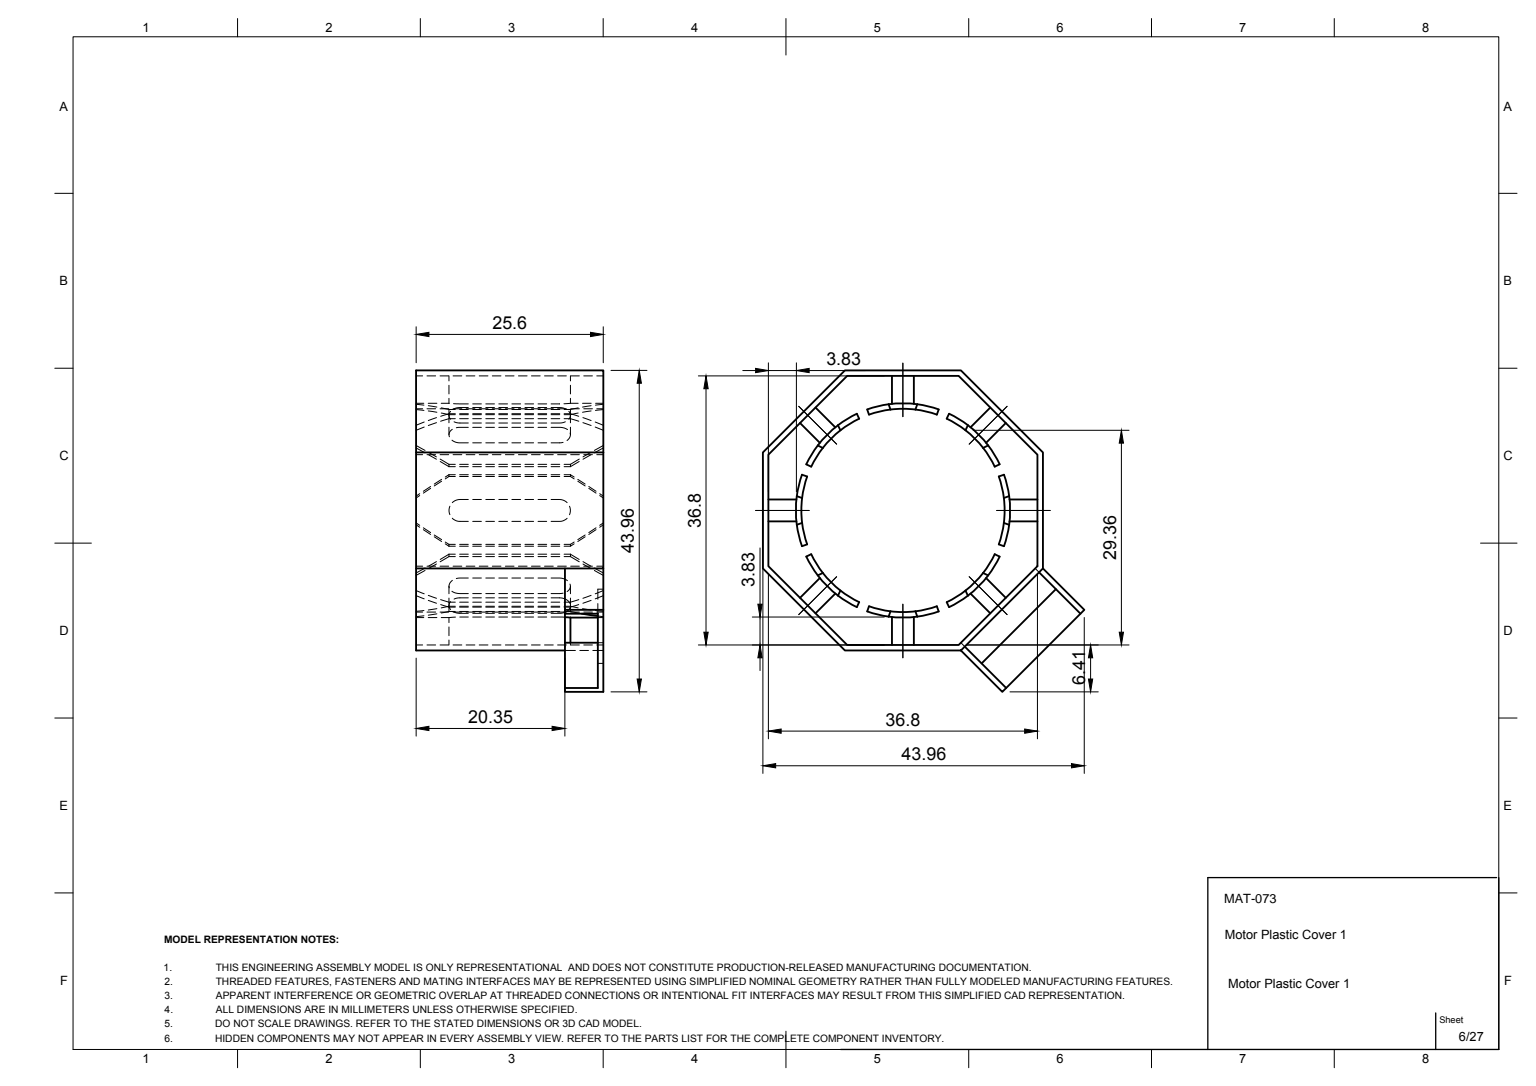
ISO-10303-21;
HEADER;
/* Generated by software containing ST-Developer
 * from STEP Tools, Inc. (www.steptools.com) 
 */

FILE_DESCRIPTION(
/* description */ ('CAx-IF Rec.Pracs.---Representation and Presentation of Product Manufa
cturing Information (PMI)---4.0---2014-10-13'),
/* implementation_level */ '2;1');

FILE_NAME(
/* name */ 'Motor Plastic Cover 1.step',
/* time_stamp */ '2026-10-24T18:52:33-07:00',
/* author */ (''),
/* organization */ (''),
/* preprocessor_version */ 'ST-DEVELOPER v20.2',
/* originating_system */ 'Autodesk Translation Framework v15.17.0.0',
/* authorisation */ '');

FILE_SCHEMA (('AP242_MANAGED_MODEL_BASED_3D_ENGINEERING_MIM_LF { 1 0 10303 442 2 1 4 }'));
ENDSEC;

DATA;
#10=MECHANICAL_DESIGN_GEOMETRIC_PRESENTATION_REPRESENTATION('',(#417),#34876);
#200=B_SPLINE_CURVE_WITH_KNOTS('',3,(#28743,#28744,#28745,#28746,#28747,
#28748,#28749,#28750,#28751,#28752,#28753,#28754,#28755,#28756,#28757,#28758,
#28759,#28760),.UNSPECIFIED.,.F.,.F.,(4,2,2,2,2,2,2,2,4),(-0.452364390465681,
-0.395818735844292,-0.339273081222902,-0.282727638227872,-0.226182195232841,
-0.16963675223781,-0.113091309242778,-0.0565456546213892,0.),
 .UNSPECIFIED.);
#201=B_SPLINE_CURVE_WITH_KNOTS('',3,(#28763,#28764,#28765,#28766,#28767,
#28768,#28769,#28770,#28771,#28772,#28773,#28774,#28775,#28776,#28777,#28778,
#28779,#28780),.UNSPECIFIED.,.F.,.F.,(4,2,2,2,2,2,2,2,4),(-0.904728780931361,
-0.848183126309972,-0.791637471688583,-0.735092028693552,-0.678546585698521,
-0.62200114270349,-0.565455699708459,-0.50891004508707,-0.452364390465681),
 .UNSPECIFIED.);
#202=B_SPLINE_CURVE_WITH_KNOTS('',3,(#28851,#28852,#28853,#28854,#28855,
#28856,#28857,#28858,#28859,#28860,#28861,#28862,#28863,#28864,#28865,#28866,
#28867,#28868),.UNSPECIFIED.,.F.,.F.,(4,2,2,2,2,2,2,2,4),(-0.452364390465681,
-0.395818735844292,-0.339273081222903,-0.282727638227872,-0.22618219523284,
-0.169636752237809,-0.113091309242778,-0.0565456546213892,0.),
 .UNSPECIFIED.);
#203=B_SPLINE_CURVE_WITH_KNOTS('',3,(#28871,#28872,#28873,#28874,#28875,
#28876,#28877,#28878,#28879,#28880,#28881,#28882,#28883,#28884,#28885,#28886,
#28887,#28888),.UNSPECIFIED.,.F.,.F.,(4,2,2,2,2,2,2,2,4),(-0.904728780931361,
-0.848183126309972,-0.791637471688583,-0.735092028693552,-0.678546585698521,
-0.622001142703489,-0.565455699708458,-0.508910045087069,-0.45236439046568),
 .UNSPECIFIED.);
#204=B_SPLINE_CURVE_WITH_KNOTS('',3,(#28959,#28960,#28961,#28962,#28963,
#28964,#28965,#28966,#28967,#28968,#28969,#28970,#28971,#28972,#28973,#28974,
#28975,#28976),.UNSPECIFIED.,.F.,.F.,(4,2,2,2,2,2,2,2,4),(-0.452364390465681,
-0.395818735844292,-0.339273081222902,-0.282727638227871,-0.22618219523284,
-0.169636752237809,-0.113091309242778,-0.0565456546213892,0.),
 .UNSPECIFIED.);
#205=B_SPLINE_CURVE_WITH_KNOTS('',3,(#28979,#28980,#28981,#28982,#28983,
#28984,#28985,#28986,#28987,#28988,#28989,#28990,#28991,#28992,#28993,#28994,
#28995,#28996),.UNSPECIFIED.,.F.,.F.,(4,2,2,2,2,2,2,2,4),(-0.904728780931362,
-0.848183126309972,-0.791637471688583,-0.735092028693552,-0.678546585698521,
-0.62200114270349,-0.565455699708459,-0.50891004508707,-0.452364390465681),
 .UNSPECIFIED.);
#206=B_SPLINE_CURVE_WITH_KNOTS('',3,(#29067,#29068,#29069,#29070,#29071,
#29072,#29073,#29074,#29075,#29076,#29077,#29078,#29079,#29080,#29081,#29082,
#29083,#29084),.UNSPECIFIED.,.F.,.F.,(4,2,2,2,2,2,2,2,4),(-0.452364390465681,
-0.395818735844292,-0.339273081222903,-0.282727638227872,-0.226182195232841,
-0.169636752237809,-0.113091309242778,-0.0565456546213892,0.),
 .UNSPECIFIED.);
#207=B_SPLINE_CURVE_WITH_KNOTS('',3,(#29087,#29088,#29089,#29090,#29091,
#29092,#29093,#29094,#29095,#29096,#29097,#29098,#29099,#29100,#29101,#29102,
#29103,#29104),.UNSPECIFIED.,.F.,.F.,(4,2,2,2,2,2,2,2,4),(-0.904728780931362,
-0.848183126309973,-0.791637471688583,-0.735092028693552,-0.678546585698521,
-0.62200114270349,-0.565455699708459,-0.50891004508707,-0.452364390465681),
 .UNSPECIFIED.);
#208=B_SPLINE_CURVE_WITH_KNOTS('',3,(#29175,#29176,#29177,#29178,#29179,
#29180,#29181,#29182,#29183,#29184,#29185,#29186,#29187,#29188,#29189,#29190,
#29191,#29192),.UNSPECIFIED.,.F.,.F.,(4,2,2,2,2,2,2,2,4),(-0.452364390465681,
-0.395818735844292,-0.339273081222903,-0.282727638227872,-0.226182195232841,
-0.169636752237809,-0.113091309242778,-0.0565456546213892,0.),
 .UNSPECIFIED.);
#209=B_SPLINE_CURVE_WITH_KNOTS('',3,(#29195,#29196,#29197,#29198,#29199,
#29200,#29201,#29202,#29203,#29204,#29205,#29206,#29207,#29208,#29209,#29210,
#29211,#29212),.UNSPECIFIED.,.F.,.F.,(4,2,2,2,2,2,2,2,4),(-0.904728780931362,
-0.848183126309973,-0.791637471688584,-0.735092028693553,-0.678546585698522,
-0.62200114270349,-0.565455699708459,-0.50891004508707,-0.452364390465681),
 .UNSPECIFIED.);
#210=B_SPLINE_CURVE_WITH_KNOTS('',3,(#29283,#29284,#29285,#29286,#29287,
#29288,#29289,#29290,#29291,#29292,#29293,#29294,#29295,#29296,#29297,#29298,
#29299,#29300),.UNSPECIFIED.,.F.,.F.,(4,2,2,2,2,2,2,2,4),(-0.452364390465681,
-0.395818735844292,-0.339273081222903,-0.282727638227872,-0.22618219523284,
-0.169636752237809,-0.113091309242778,-0.0565456546213891,0.),
 .UNSPECIFIED.);
#211=B_SPLINE_CURVE_WITH_KNOTS('',3,(#29303,#29304,#29305,#29306,#29307,
#29308,#29309,#29310,#29311,#29312,#29313,#29314,#29315,#29316,#29317,#29318,
#29319,#29320),.UNSPECIFIED.,.F.,.F.,(4,2,2,2,2,2,2,2,4),(-0.904728780931362,
-0.848183126309973,-0.791637471688583,-0.735092028693552,-0.678546585698521,
-0.62200114270349,-0.565455699708459,-0.50891004508707,-0.452364390465681),
 .UNSPECIFIED.);
#212=B_SPLINE_CURVE_WITH_KNOTS('',3,(#29391,#29392,#29393,#29394,#29395,
#29396,#29397,#29398,#29399,#29400,#29401,#29402,#29403,#29404,#29405,#29406,
#29407,#29408),.UNSPECIFIED.,.F.,.F.,(4,2,2,2,2,2,2,2,4),(-0.452364390465681,
-0.395818735844292,-0.339273081222902,-0.282727638227872,-0.226182195232841,
-0.169636752237809,-0.113091309242778,-0.0565456546213892,0.),
 .UNSPECIFIED.);
#213=B_SPLINE_CURVE_WITH_KNOTS('',3,(#29411,#29412,#29413,#29414,#29415,
#29416,#29417,#29418,#29419,#29420,#29421,#29422,#29423,#29424,#29425,#29426,
#29427,#29428),.UNSPECIFIED.,.F.,.F.,(4,2,2,2,2,2,2,2,4),(-0.904728780931362,
-0.848183126309973,-0.791637471688583,-0.735092028693552,-0.678546585698521,
-0.62200114270349,-0.565455699708459,-0.50891004508707,-0.452364390465681),
 .UNSPECIFIED.);
#214=B_SPLINE_CURVE_WITH_KNOTS('',3,(#29499,#29500,#29501,#29502,#29503,
#29504,#29505,#29506,#29507,#29508,#29509,#29510,#29511,#29512,#29513,#29514,
#29515,#29516),.UNSPECIFIED.,.F.,.F.,(4,2,2,2,2,2,2,2,4),(-0.452364390465681,
-0.395818735844292,-0.339273081222903,-0.282727638227872,-0.226182195232841,
-0.169636752237809,-0.113091309242778,-0.0565456546213892,0.),
 .UNSPECIFIED.);
#215=B_SPLINE_CURVE_WITH_KNOTS('',3,(#29519,#29520,#29521,#29522,#29523,
#29524,#29525,#29526,#29527,#29528,#29529,#29530,#29531,#29532,#29533,#29534,
#29535,#29536),.UNSPECIFIED.,.F.,.F.,(4,2,2,2,2,2,2,2,4),(-0.904728780931362,
-0.848183126309973,-0.791637471688583,-0.735092028693552,-0.678546585698521,
-0.62200114270349,-0.565455699708459,-0.50891004508707,-0.452364390465681),
 .UNSPECIFIED.);
#236=ELLIPSE('',#20061,0.0264106630927894,0.0146500000000133);
#237=ELLIPSE('',#20063,0.0264106630927895,0.0146500000000133);
#238=ELLIPSE('',#20064,0.0264106630927895,0.0146500000000133);
#239=ELLIPSE('',#20066,0.0264106630927894,0.0146500000000133);
#240=ELLIPSE('',#20069,0.0250585813644904,0.0139000000000133);
#241=ELLIPSE('',#20073,0.0250585813644904,0.0139000000000133);
#242=ELLIPSE('',#20076,0.0250585813644904,0.0139000000000133);
#243=ELLIPSE('',#20078,0.0250585813644904,0.0139000000000133);
#244=ELLIPSE('',#20089,0.0264106630927891,0.0146500000000128);
#245=ELLIPSE('',#20091,0.0264106630927891,0.0146500000000128);
#246=ELLIPSE('',#20092,0.0264106630927891,0.0146500000000128);
#247=ELLIPSE('',#20094,0.0264106630927891,0.0146500000000128);
#248=ELLIPSE('',#20097,0.0250585813644901,0.0139000000000128);
#249=ELLIPSE('',#20101,0.0250585813644901,0.0139000000000128);
#250=ELLIPSE('',#20104,0.0250585813644901,0.0139000000000128);
#251=ELLIPSE('',#20106,0.0250585813644901,0.0139000000000128);
#252=ELLIPSE('',#20117,0.0264106630927895,0.0146500000000133);
#253=ELLIPSE('',#20119,0.0264106630927894,0.0146500000000133);
#254=ELLIPSE('',#20120,0.0264106630927894,0.0146500000000133);
#255=ELLIPSE('',#20122,0.0264106630927895,0.0146500000000133);
#256=ELLIPSE('',#20125,0.0250585813644904,0.0139000000000133);
#257=ELLIPSE('',#20129,0.0250585813644904,0.0139000000000133);
#258=ELLIPSE('',#20132,0.0250585813644904,0.0139000000000133);
#259=ELLIPSE('',#20134,0.0250585813644904,0.0139000000000133);
#260=ELLIPSE('',#20145,0.0264106630927891,0.0146500000000128);
#261=ELLIPSE('',#20147,0.0264106630927891,0.0146500000000128);
#262=ELLIPSE('',#20148,0.0264106630927891,0.0146500000000128);
#263=ELLIPSE('',#20150,0.0264106630927891,0.0146500000000128);
#264=ELLIPSE('',#20153,0.0250585813644901,0.0139000000000128);
#265=ELLIPSE('',#20157,0.0250585813644901,0.0139000000000128);
#266=ELLIPSE('',#20160,0.0250585813644901,0.0139000000000128);
#267=ELLIPSE('',#20162,0.0250585813644901,0.0139000000000128);
#268=ELLIPSE('',#20173,0.0264106630927894,0.0146500000000133);
#269=ELLIPSE('',#20175,0.0264106630927895,0.0146500000000133);
#270=ELLIPSE('',#20176,0.0264106630927894,0.0146500000000133);
#271=ELLIPSE('',#20178,0.0264106630927894,0.0146500000000133);
#272=ELLIPSE('',#20181,0.0250585813644904,0.0139000000000133);
#273=ELLIPSE('',#20185,0.0250585813644904,0.0139000000000133);
#274=ELLIPSE('',#20188,0.0250585813644904,0.0139000000000133);
#275=ELLIPSE('',#20190,0.0250585813644904,0.0139000000000133);
#276=ELLIPSE('',#20201,0.0264106630927891,0.0146500000000128);
#277=ELLIPSE('',#20203,0.0264106630927891,0.0146500000000128);
#278=ELLIPSE('',#20204,0.0264106630927891,0.0146500000000128);
#279=ELLIPSE('',#20206,0.0264106630927891,0.0146500000000128);
#280=ELLIPSE('',#20209,0.0250585813644901,0.0139000000000128);
#281=ELLIPSE('',#20213,0.0250585813644901,0.0139000000000128);
#282=ELLIPSE('',#20216,0.0250585813644901,0.0139000000000128);
#283=ELLIPSE('',#20218,0.0250585813644901,0.0139000000000128);
#284=ELLIPSE('',#20229,0.0264106630927895,0.0146500000000133);
#285=ELLIPSE('',#20231,0.0264106630927894,0.0146500000000133);
#286=ELLIPSE('',#20232,0.0264106630927894,0.0146500000000133);
#287=ELLIPSE('',#20234,0.0264106630927895,0.0146500000000133);
#288=ELLIPSE('',#20237,0.0250585813644904,0.0139000000000133);
#289=ELLIPSE('',#20241,0.0250585813644904,0.0139000000000133);
#290=ELLIPSE('',#20244,0.0250585813644904,0.0139000000000133);
#291=ELLIPSE('',#20246,0.0250585813644904,0.0139000000000133);
#292=ELLIPSE('',#20257,0.0264106630927891,0.0146500000000128);
#293=ELLIPSE('',#20259,0.0264106630927891,0.0146500000000128);
#294=ELLIPSE('',#20260,0.0264106630927891,0.0146500000000128);
#295=ELLIPSE('',#20262,0.0264106630927891,0.0146500000000128);
#296=ELLIPSE('',#20265,0.0250585813644901,0.0139000000000128);
#297=ELLIPSE('',#20269,0.0250585813644901,0.0139000000000128);
#298=ELLIPSE('',#20272,0.0250585813644901,0.0139000000000128);
#299=ELLIPSE('',#20274,0.0250585813644901,0.0139000000000128);
#351=SHAPE_REPRESENTATION_RELATIONSHIP('SRR','None',#34988,#384);
#384=ADVANCED_BREP_SHAPE_REPRESENTATION('',(#450),#34846);
#417=STYLED_ITEM('',(#35162),#450);
#450=MANIFOLD_SOLID_BREP('Motor Plastic Cover 1',#19557);
#484=FACE_BOUND('',#5889,.T.);
#485=FACE_BOUND('',#5904,.T.);
#486=FACE_BOUND('',#5919,.T.);
#487=FACE_BOUND('',#5934,.T.);
#488=FACE_BOUND('',#5949,.T.);
#489=FACE_BOUND('',#5964,.T.);
#490=FACE_BOUND('',#5979,.T.);
#491=FACE_BOUND('',#5994,.T.);
#492=FACE_BOUND('',#6009,.T.);
#493=FACE_BOUND('',#6018,.T.);
#494=FACE_BOUND('',#6020,.T.);
#495=FACE_BOUND('',#6022,.T.);
#496=FACE_BOUND('',#6024,.T.);
#497=FACE_BOUND('',#6026,.T.);
#498=FACE_BOUND('',#6028,.T.);
#499=FACE_BOUND('',#6030,.T.);
#500=FACE_BOUND('',#6032,.T.);
#608=PLANE('',#20067);
#609=PLANE('',#20068);
#610=PLANE('',#20070);
#611=PLANE('',#20072);
#612=PLANE('',#20074);
#613=PLANE('',#20075);
#614=PLANE('',#20080);
#615=PLANE('',#20081);
#616=PLANE('',#20082);
#617=PLANE('',#20087);
#618=PLANE('',#20095);
#619=PLANE('',#20096);
#620=PLANE('',#20098);
#621=PLANE('',#20100);
#622=PLANE('',#20102);
#623=PLANE('',#20103);
#624=PLANE('',#20108);
#625=PLANE('',#20109);
#626=PLANE('',#20110);
#627=PLANE('',#20115);
#628=PLANE('',#20123);
#629=PLANE('',#20124);
#630=PLANE('',#20126);
#631=PLANE('',#20128);
#632=PLANE('',#20130);
#633=PLANE('',#20131);
#634=PLANE('',#20136);
#635=PLANE('',#20137);
#636=PLANE('',#20138);
#637=PLANE('',#20143);
#638=PLANE('',#20151);
#639=PLANE('',#20152);
#640=PLANE('',#20154);
#641=PLANE('',#20156);
#642=PLANE('',#20158);
#643=PLANE('',#20159);
#644=PLANE('',#20164);
#645=PLANE('',#20165);
#646=PLANE('',#20166);
#647=PLANE('',#20171);
#648=PLANE('',#20179);
#649=PLANE('',#20180);
#650=PLANE('',#20182);
#651=PLANE('',#20184);
#652=PLANE('',#20186);
#653=PLANE('',#20187);
#654=PLANE('',#20192);
#655=PLANE('',#20193);
#656=PLANE('',#20194);
#657=PLANE('',#20199);
#658=PLANE('',#20207);
#659=PLANE('',#20208);
#660=PLANE('',#20210);
#661=PLANE('',#20212);
#662=PLANE('',#20214);
#663=PLANE('',#20215);
#664=PLANE('',#20220);
#665=PLANE('',#20221);
#666=PLANE('',#20222);
#667=PLANE('',#20227);
#668=PLANE('',#20235);
#669=PLANE('',#20236);
#670=PLANE('',#20238);
#671=PLANE('',#20240);
#672=PLANE('',#20242);
#673=PLANE('',#20243);
#674=PLANE('',#20248);
#675=PLANE('',#20249);
#676=PLANE('',#20250);
#677=PLANE('',#20255);
#678=PLANE('',#20263);
#679=PLANE('',#20264);
#680=PLANE('',#20266);
#681=PLANE('',#20268);
#682=PLANE('',#20270);
#683=PLANE('',#20271);
#684=PLANE('',#20276);
#685=PLANE('',#20277);
#686=PLANE('',#20278);
#687=PLANE('',#20285);
#688=PLANE('',#20286);
#689=PLANE('',#20287);
#690=PLANE('',#20288);
#691=PLANE('',#20289);
#692=PLANE('',#20290);
#693=PLANE('',#20291);
#694=PLANE('',#20292);
#695=PLANE('',#20293);
#696=PLANE('',#20294);
#697=PLANE('',#20295);
#698=PLANE('',#20296);
#699=PLANE('',#20297);
#700=PLANE('',#20298);
#701=PLANE('',#20299);
#702=PLANE('',#20300);
#703=PLANE('',#20301);
#704=PLANE('',#20302);
#705=PLANE('',#20303);
#706=PLANE('',#20304);
#707=PLANE('',#20305);
#708=PLANE('',#20306);
#709=PLANE('',#20307);
#710=PLANE('',#20308);
#711=PLANE('',#20309);
#712=PLANE('',#20310);
#713=PLANE('',#20311);
#714=PLANE('',#20312);
#715=PLANE('',#20313);
#716=PLANE('',#20314);
#1145=LINE('',#28731,#2744);
#1146=LINE('',#28738,#2745);
#1147=LINE('',#28741,#2746);
#1148=LINE('',#28762,#2747);
#1149=LINE('',#28783,#2748);
#1150=LINE('',#28785,#2749);
#1151=LINE('',#28786,#2750);
#1152=LINE('',#28789,#2751);
#1153=LINE('',#28793,#2752);
#1154=LINE('',#28798,#2753);
#1155=LINE('',#28801,#2754);
#1156=LINE('',#28802,#2755);
#1157=LINE('',#28805,#2756);
#1158=LINE('',#28812,#2757);
#1159=LINE('',#28816,#2758);
#1160=LINE('',#28818,#2759);
#1161=LINE('',#28819,#2760);
#1162=LINE('',#28822,#2761);
#1163=LINE('',#28827,#2762);
#1164=LINE('',#28829,#2763);
#1165=LINE('',#28839,#2764);
#1166=LINE('',#28846,#2765);
#1167=LINE('',#28849,#2766);
#1168=LINE('',#28870,#2767);
#1169=LINE('',#28891,#2768);
#1170=LINE('',#28893,#2769);
#1171=LINE('',#28894,#2770);
#1172=LINE('',#28897,#2771);
#1173=LINE('',#28901,#2772);
#1174=LINE('',#28906,#2773);
#1175=LINE('',#28909,#2774);
#1176=LINE('',#28910,#2775);
#1177=LINE('',#28913,#2776);
#1178=LINE('',#28920,#2777);
#1179=LINE('',#28924,#2778);
#1180=LINE('',#28926,#2779);
#1181=LINE('',#28927,#2780);
#1182=LINE('',#28930,#2781);
#1183=LINE('',#28935,#2782);
#1184=LINE('',#28937,#2783);
#1185=LINE('',#28947,#2784);
#1186=LINE('',#28954,#2785);
#1187=LINE('',#28957,#2786);
#1188=LINE('',#28978,#2787);
#1189=LINE('',#28999,#2788);
#1190=LINE('',#29001,#2789);
#1191=LINE('',#29002,#2790);
#1192=LINE('',#29005,#2791);
#1193=LINE('',#29009,#2792);
#1194=LINE('',#29014,#2793);
#1195=LINE('',#29017,#2794);
#1196=LINE('',#29018,#2795);
#1197=LINE('',#29021,#2796);
#1198=LINE('',#29028,#2797);
#1199=LINE('',#29032,#2798);
#1200=LINE('',#29034,#2799);
#1201=LINE('',#29035,#2800);
#1202=LINE('',#29038,#2801);
#1203=LINE('',#29043,#2802);
#1204=LINE('',#29045,#2803);
#1205=LINE('',#29055,#2804);
#1206=LINE('',#29062,#2805);
#1207=LINE('',#29065,#2806);
#1208=LINE('',#29086,#2807);
#1209=LINE('',#29107,#2808);
#1210=LINE('',#29109,#2809);
#1211=LINE('',#29110,#2810);
#1212=LINE('',#29113,#2811);
#1213=LINE('',#29117,#2812);
#1214=LINE('',#29122,#2813);
#1215=LINE('',#29125,#2814);
#1216=LINE('',#29126,#2815);
#1217=LINE('',#29129,#2816);
#1218=LINE('',#29136,#2817);
#1219=LINE('',#29140,#2818);
#1220=LINE('',#29142,#2819);
#1221=LINE('',#29143,#2820);
#1222=LINE('',#29146,#2821);
#1223=LINE('',#29151,#2822);
#1224=LINE('',#29153,#2823);
#1225=LINE('',#29163,#2824);
#1226=LINE('',#29170,#2825);
#1227=LINE('',#29173,#2826);
#1228=LINE('',#29194,#2827);
#1229=LINE('',#29215,#2828);
#1230=LINE('',#29217,#2829);
#1231=LINE('',#29218,#2830);
#1232=LINE('',#29221,#2831);
#1233=LINE('',#29225,#2832);
#1234=LINE('',#29230,#2833);
#1235=LINE('',#29233,#2834);
#1236=LINE('',#29234,#2835);
#1237=LINE('',#29237,#2836);
#1238=LINE('',#29244,#2837);
#1239=LINE('',#29248,#2838);
#1240=LINE('',#29250,#2839);
#1241=LINE('',#29251,#2840);
#1242=LINE('',#29254,#2841);
#1243=LINE('',#29259,#2842);
#1244=LINE('',#29261,#2843);
#1245=LINE('',#29271,#2844);
#1246=LINE('',#29278,#2845);
#1247=LINE('',#29281,#2846);
#1248=LINE('',#29302,#2847);
#1249=LINE('',#29323,#2848);
#1250=LINE('',#29325,#2849);
#1251=LINE('',#29326,#2850);
#1252=LINE('',#29329,#2851);
#1253=LINE('',#29333,#2852);
#1254=LINE('',#29338,#2853);
#1255=LINE('',#29341,#2854);
#1256=LINE('',#29342,#2855);
#1257=LINE('',#29345,#2856);
#1258=LINE('',#29352,#2857);
#1259=LINE('',#29356,#2858);
#1260=LINE('',#29358,#2859);
#1261=LINE('',#29359,#2860);
#1262=LINE('',#29362,#2861);
#1263=LINE('',#29367,#2862);
#1264=LINE('',#29369,#2863);
#1265=LINE('',#29379,#2864);
#1266=LINE('',#29386,#2865);
#1267=LINE('',#29389,#2866);
#1268=LINE('',#29410,#2867);
#1269=LINE('',#29431,#2868);
#1270=LINE('',#29433,#2869);
#1271=LINE('',#29434,#2870);
#1272=LINE('',#29437,#2871);
#1273=LINE('',#29441,#2872);
#1274=LINE('',#29446,#2873);
#1275=LINE('',#29449,#2874);
#1276=LINE('',#29450,#2875);
#1277=LINE('',#29453,#2876);
#1278=LINE('',#29460,#2877);
#1279=LINE('',#29464,#2878);
#1280=LINE('',#29466,#2879);
#1281=LINE('',#29467,#2880);
#1282=LINE('',#29470,#2881);
#1283=LINE('',#29475,#2882);
#1284=LINE('',#29477,#2883);
#1285=LINE('',#29487,#2884);
#1286=LINE('',#29494,#2885);
#1287=LINE('',#29497,#2886);
#1288=LINE('',#29518,#2887);
#1289=LINE('',#29539,#2888);
#1290=LINE('',#29541,#2889);
#1291=LINE('',#29542,#2890);
#1292=LINE('',#29545,#2891);
#1293=LINE('',#29549,#2892);
#1294=LINE('',#29554,#2893);
#1295=LINE('',#29557,#2894);
#1296=LINE('',#29558,#2895);
#1297=LINE('',#29561,#2896);
#1298=LINE('',#29568,#2897);
#1299=LINE('',#29572,#2898);
#1300=LINE('',#29574,#2899);
#1301=LINE('',#29575,#2900);
#1302=LINE('',#29578,#2901);
#1303=LINE('',#29587,#2902);
#1304=LINE('',#29589,#2903);
#1305=LINE('',#29593,#2904);
#1306=LINE('',#29595,#2905);
#1307=LINE('',#29597,#2906);
#1308=LINE('',#29599,#2907);
#1309=LINE('',#29601,#2908);
#1310=LINE('',#29603,#2909);
#1311=LINE('',#29605,#2910);
#1312=LINE('',#29606,#2911);
#1313=LINE('',#29609,#2912);
#1314=LINE('',#29611,#2913);
#1315=LINE('',#29613,#2914);
#1316=LINE('',#29615,#2915);
#1317=LINE('',#29617,#2916);
#1318=LINE('',#29619,#2917);
#1319=LINE('',#29621,#2918);
#1320=LINE('',#29622,#2919);
#1321=LINE('',#29625,#2920);
#1322=LINE('',#29627,#2921);
#1323=LINE('',#29628,#2922);
#1324=LINE('',#29631,#2923);
#1325=LINE('',#29632,#2924);
#1326=LINE('',#29636,#2925);
#1327=LINE('',#29637,#2926);
#1328=LINE('',#29638,#2927);
#1329=LINE('',#29641,#2928);
#1330=LINE('',#29643,#2929);
#1331=LINE('',#29645,#2930);
#1332=LINE('',#29646,#2931);
#1333=LINE('',#29649,#2932);
#1334=LINE('',#29650,#2933);
#1335=LINE('',#29653,#2934);
#1336=LINE('',#29654,#2935);
#1337=LINE('',#29656,#2936);
#1338=LINE('',#29659,#2937);
#1339=LINE('',#29661,#2938);
#1340=LINE('',#29662,#2939);
#1341=LINE('',#29665,#2940);
#1342=LINE('',#29667,#2941);
#1343=LINE('',#29669,#2942);
#1344=LINE('',#29671,#2943);
#1345=LINE('',#29673,#2944);
#1346=LINE('',#29675,#2945);
#1347=LINE('',#29677,#2946);
#1348=LINE('',#29679,#2947);
#1349=LINE('',#29681,#2948);
#1350=LINE('',#29683,#2949);
#1351=LINE('',#29685,#2950);
#1352=LINE('',#29686,#2951);
#1353=LINE('',#29688,#2952);
#1354=LINE('',#29689,#2953);
#1355=LINE('',#29691,#2954);
#1356=LINE('',#29693,#2955);
#1357=LINE('',#29695,#2956);
#1358=LINE('',#29697,#2957);
#1359=LINE('',#29699,#2958);
#1360=LINE('',#29701,#2959);
#1361=LINE('',#29704,#2960);
#1362=LINE('',#29706,#2961);
#1363=LINE('',#29708,#2962);
#1364=LINE('',#29710,#2963);
#1365=LINE('',#29711,#2964);
#1366=LINE('',#29712,#2965);
#1367=LINE('',#29716,#2966);
#1368=LINE('',#29718,#2967);
#1369=LINE('',#29719,#2968);
#1370=LINE('',#29720,#2969);
#1371=LINE('',#29721,#2970);
#1372=LINE('',#29724,#2971);
#1373=LINE('',#29726,#2972);
#1374=LINE('',#29728,#2973);
#1375=LINE('',#29729,#2974);
#1376=LINE('',#29730,#2975);
#1377=LINE('',#29734,#2976);
#1378=LINE('',#29735,#2977);
#1379=LINE('',#29737,#2978);
#1380=LINE('',#29738,#2979);
#1381=LINE('',#29739,#2980);
#1382=LINE('',#29741,#2981);
#1383=LINE('',#29742,#2982);
#1384=LINE('',#29744,#2983);
#1385=LINE('',#29745,#2984);
#1386=LINE('',#29751,#2985);
#2744=VECTOR('',#22546,1.);
#2745=VECTOR('',#22553,1.);
#2746=VECTOR('',#22554,1.);
#2747=VECTOR('',#22555,1.);
#2748=VECTOR('',#22558,1.);
#2749=VECTOR('',#22559,1.);
#2750=VECTOR('',#22560,1.);
#2751=VECTOR('',#22563,1.);
#2752=VECTOR('',#22568,1.);
#2753=VECTOR('',#22575,1.);
#2754=VECTOR('',#22578,1.);
#2755=VECTOR('',#22579,1.);
#2756=VECTOR('',#22582,1.);
#2757=VECTOR('',#22593,1.);
#2758=VECTOR('',#22598,1.);
#2759=VECTOR('',#22599,1.);
#2760=VECTOR('',#22600,1.);
#2761=VECTOR('',#22603,1.);
#2762=VECTOR('',#22610,1.);
#2763=VECTOR('',#22613,1.);
#2764=VECTOR('',#22622,1.);
#2765=VECTOR('',#22629,1.);
#2766=VECTOR('',#22630,1.);
#2767=VECTOR('',#22631,1.);
#2768=VECTOR('',#22634,1.);
#2769=VECTOR('',#22635,1.);
#2770=VECTOR('',#22636,1.);
#2771=VECTOR('',#22639,1.);
#2772=VECTOR('',#22644,1.);
#2773=VECTOR('',#22651,1.);
#2774=VECTOR('',#22654,1.);
#2775=VECTOR('',#22655,1.);
#2776=VECTOR('',#22658,1.);
#2777=VECTOR('',#22669,1.);
#2778=VECTOR('',#22674,1.);
#2779=VECTOR('',#22675,1.);
#2780=VECTOR('',#22676,1.);
#2781=VECTOR('',#22679,1.);
#2782=VECTOR('',#22686,1.);
#2783=VECTOR('',#22689,1.);
#2784=VECTOR('',#22698,1.);
#2785=VECTOR('',#22705,1.);
#2786=VECTOR('',#22706,1.);
#2787=VECTOR('',#22707,1.);
#2788=VECTOR('',#22710,1.);
#2789=VECTOR('',#22711,1.);
#2790=VECTOR('',#22712,1.);
#2791=VECTOR('',#22715,1.);
#2792=VECTOR('',#22720,1.);
#2793=VECTOR('',#22727,1.);
#2794=VECTOR('',#22730,1.);
#2795=VECTOR('',#22731,1.);
#2796=VECTOR('',#22734,1.);
#2797=VECTOR('',#22745,1.);
#2798=VECTOR('',#22750,1.);
#2799=VECTOR('',#22751,1.);
#2800=VECTOR('',#22752,1.);
#2801=VECTOR('',#22755,1.);
#2802=VECTOR('',#22762,1.);
#2803=VECTOR('',#22765,1.);
#2804=VECTOR('',#22774,1.);
#2805=VECTOR('',#22781,1.);
#2806=VECTOR('',#22782,1.);
#2807=VECTOR('',#22783,1.);
#2808=VECTOR('',#22786,1.);
#2809=VECTOR('',#22787,1.);
#2810=VECTOR('',#22788,1.);
#2811=VECTOR('',#22791,1.);
#2812=VECTOR('',#22796,1.);
#2813=VECTOR('',#22803,1.);
#2814=VECTOR('',#22806,1.);
#2815=VECTOR('',#22807,1.);
#2816=VECTOR('',#22810,1.);
#2817=VECTOR('',#22821,1.);
#2818=VECTOR('',#22826,1.);
#2819=VECTOR('',#22827,1.);
#2820=VECTOR('',#22828,1.);
#2821=VECTOR('',#22831,1.);
#2822=VECTOR('',#22838,1.);
#2823=VECTOR('',#22841,1.);
#2824=VECTOR('',#22850,1.);
#2825=VECTOR('',#22857,1.);
#2826=VECTOR('',#22858,1.);
#2827=VECTOR('',#22859,1.);
#2828=VECTOR('',#22862,1.);
#2829=VECTOR('',#22863,1.);
#2830=VECTOR('',#22864,1.);
#2831=VECTOR('',#22867,1.);
#2832=VECTOR('',#22872,1.);
#2833=VECTOR('',#22879,1.);
#2834=VECTOR('',#22882,1.);
#2835=VECTOR('',#22883,1.);
#2836=VECTOR('',#22886,1.);
#2837=VECTOR('',#22897,1.);
#2838=VECTOR('',#22902,1.);
#2839=VECTOR('',#22903,1.);
#2840=VECTOR('',#22904,1.);
#2841=VECTOR('',#22907,1.);
#2842=VECTOR('',#22914,1.);
#2843=VECTOR('',#22917,1.);
#2844=VECTOR('',#22926,1.);
#2845=VECTOR('',#22933,1.);
#2846=VECTOR('',#22934,1.);
#2847=VECTOR('',#22935,1.);
#2848=VECTOR('',#22938,1.);
#2849=VECTOR('',#22939,1.);
#2850=VECTOR('',#22940,1.);
#2851=VECTOR('',#22943,1.);
#2852=VECTOR('',#22948,1.);
#2853=VECTOR('',#22955,1.);
#2854=VECTOR('',#22958,1.);
#2855=VECTOR('',#22959,1.);
#2856=VECTOR('',#22962,1.);
#2857=VECTOR('',#22973,1.);
#2858=VECTOR('',#22978,1.);
#2859=VECTOR('',#22979,1.);
#2860=VECTOR('',#22980,1.);
#2861=VECTOR('',#22983,1.);
#2862=VECTOR('',#22990,1.);
#2863=VECTOR('',#22993,1.);
#2864=VECTOR('',#23002,1.);
#2865=VECTOR('',#23009,1.);
#2866=VECTOR('',#23010,1.);
#2867=VECTOR('',#23011,1.);
#2868=VECTOR('',#23014,1.);
#2869=VECTOR('',#23015,1.);
#2870=VECTOR('',#23016,1.);
#2871=VECTOR('',#23019,1.);
#2872=VECTOR('',#23024,1.);
#2873=VECTOR('',#23031,1.);
#2874=VECTOR('',#23034,1.);
#2875=VECTOR('',#23035,1.);
#2876=VECTOR('',#23038,1.);
#2877=VECTOR('',#23049,1.);
#2878=VECTOR('',#23054,1.);
#2879=VECTOR('',#23055,1.);
#2880=VECTOR('',#23056,1.);
#2881=VECTOR('',#23059,1.);
#2882=VECTOR('',#23066,1.);
#2883=VECTOR('',#23069,1.);
#2884=VECTOR('',#23078,1.);
#2885=VECTOR('',#23085,1.);
#2886=VECTOR('',#23086,1.);
#2887=VECTOR('',#23087,1.);
#2888=VECTOR('',#23090,1.);
#2889=VECTOR('',#23091,1.);
#2890=VECTOR('',#23092,1.);
#2891=VECTOR('',#23095,1.);
#2892=VECTOR('',#23100,1.);
#2893=VECTOR('',#23107,1.);
#2894=VECTOR('',#23110,1.);
#2895=VECTOR('',#23111,1.);
#2896=VECTOR('',#23114,1.);
#2897=VECTOR('',#23125,1.);
#2898=VECTOR('',#23130,1.);
#2899=VECTOR('',#23131,1.);
#2900=VECTOR('',#23132,1.);
#2901=VECTOR('',#23135,1.);
#2902=VECTOR('',#23146,1.);
#2903=VECTOR('',#23149,1.);
#2904=VECTOR('',#23152,1.);
#2905=VECTOR('',#23153,1.);
#2906=VECTOR('',#23154,1.);
#2907=VECTOR('',#23155,1.);
#2908=VECTOR('',#23156,1.);
#2909=VECTOR('',#23157,1.);
#2910=VECTOR('',#23158,1.);
#2911=VECTOR('',#23159,1.);
#2912=VECTOR('',#23160,1.);
#2913=VECTOR('',#23161,1.);
#2914=VECTOR('',#23162,1.);
#2915=VECTOR('',#23163,1.);
#2916=VECTOR('',#23164,1.);
#2917=VECTOR('',#23165,1.);
#2918=VECTOR('',#23166,1.);
#2919=VECTOR('',#23167,1.);
#2920=VECTOR('',#23170,1.);
#2921=VECTOR('',#23171,1.);
#2922=VECTOR('',#23172,1.);
#2923=VECTOR('',#23175,1.);
#2924=VECTOR('',#23176,1.);
#2925=VECTOR('',#23179,1.);
#2926=VECTOR('',#23180,1.);
#2927=VECTOR('',#23181,1.);
#2928=VECTOR('',#23184,1.);
#2929=VECTOR('',#23185,1.);
#2930=VECTOR('',#23186,1.);
#2931=VECTOR('',#23187,1.);
#2932=VECTOR('',#23190,1.);
#2933=VECTOR('',#23191,1.);
#2934=VECTOR('',#23194,1.);
#2935=VECTOR('',#23195,1.);
#2936=VECTOR('',#23198,1.);
#2937=VECTOR('',#23201,1.);
#2938=VECTOR('',#23202,1.);
#2939=VECTOR('',#23203,1.);
#2940=VECTOR('',#23204,1.);
#2941=VECTOR('',#23205,1.);
#2942=VECTOR('',#23206,1.);
#2943=VECTOR('',#23207,1.);
#2944=VECTOR('',#23208,1.);
#2945=VECTOR('',#23209,1.);
#2946=VECTOR('',#23210,1.);
#2947=VECTOR('',#23211,1.);
#2948=VECTOR('',#23212,1.);
#2949=VECTOR('',#23213,1.);
#2950=VECTOR('',#23214,1.);
#2951=VECTOR('',#23215,1.);
#2952=VECTOR('',#23218,1.);
#2953=VECTOR('',#23219,1.);
#2954=VECTOR('',#23222,1.);
#2955=VECTOR('',#23225,1.);
#2956=VECTOR('',#23228,1.);
#2957=VECTOR('',#23231,1.);
#2958=VECTOR('',#23234,1.);
#2959=VECTOR('',#23237,1.);
#2960=VECTOR('',#23240,1.);
#2961=VECTOR('',#23241,1.);
#2962=VECTOR('',#23242,1.);
#2963=VECTOR('',#23243,1.);
#2964=VECTOR('',#23244,1.);
#2965=VECTOR('',#23245,1.);
#2966=VECTOR('',#23248,1.);
#2967=VECTOR('',#23249,1.);
#2968=VECTOR('',#23250,1.);
#2969=VECTOR('',#23251,1.);
#2970=VECTOR('',#23252,1.);
#2971=VECTOR('',#23255,1.);
#2972=VECTOR('',#23256,1.);
#2973=VECTOR('',#23257,1.);
#2974=VECTOR('',#23258,1.);
#2975=VECTOR('',#23259,1.);
#2976=VECTOR('',#23264,1.);
#2977=VECTOR('',#23265,1.);
#2978=VECTOR('',#23266,1.);
#2979=VECTOR('',#23267,1.);
#2980=VECTOR('',#23268,1.);
#2981=VECTOR('',#23271,1.);
#2982=VECTOR('',#23272,1.);
#2983=VECTOR('',#23275,1.);
#2984=VECTOR('',#23276,1.);
#2985=VECTOR('',#23287,1.);
#4307=CYLINDRICAL_SURFACE('',#20060,0.01465);
#4308=CYLINDRICAL_SURFACE('',#20077,0.0139);
#4309=CYLINDRICAL_SURFACE('',#20083,0.0015);
#4310=CYLINDRICAL_SURFACE('',#20085,0.0015);
#4311=CYLINDRICAL_SURFACE('',#20088,0.01465);
#4312=CYLINDRICAL_SURFACE('',#20105,0.0139);
#4313=CYLINDRICAL_SURFACE('',#20111,0.0015);
#4314=CYLINDRICAL_SURFACE('',#20113,0.0015);
#4315=CYLINDRICAL_SURFACE('',#20116,0.01465);
#4316=CYLINDRICAL_SURFACE('',#20133,0.0139);
#4317=CYLINDRICAL_SURFACE('',#20139,0.0015);
#4318=CYLINDRICAL_SURFACE('',#20141,0.0015);
#4319=CYLINDRICAL_SURFACE('',#20144,0.01465);
#4320=CYLINDRICAL_SURFACE('',#20161,0.0139);
#4321=CYLINDRICAL_SURFACE('',#20167,0.0015);
#4322=CYLINDRICAL_SURFACE('',#20169,0.0015);
#4323=CYLINDRICAL_SURFACE('',#20172,0.01465);
#4324=CYLINDRICAL_SURFACE('',#20189,0.0139);
#4325=CYLINDRICAL_SURFACE('',#20195,0.0015);
#4326=CYLINDRICAL_SURFACE('',#20197,0.0015);
#4327=CYLINDRICAL_SURFACE('',#20200,0.01465);
#4328=CYLINDRICAL_SURFACE('',#20217,0.0139);
#4329=CYLINDRICAL_SURFACE('',#20223,0.0015);
#4330=CYLINDRICAL_SURFACE('',#20225,0.0015);
#4331=CYLINDRICAL_SURFACE('',#20228,0.01465);
#4332=CYLINDRICAL_SURFACE('',#20245,0.0139);
#4333=CYLINDRICAL_SURFACE('',#20251,0.0015);
#4334=CYLINDRICAL_SURFACE('',#20253,0.0015);
#4335=CYLINDRICAL_SURFACE('',#20256,0.01465);
#4336=CYLINDRICAL_SURFACE('',#20273,0.0139);
#4337=CYLINDRICAL_SURFACE('',#20279,0.0015);
#4338=CYLINDRICAL_SURFACE('',#20281,0.0015);
#4839=FACE_OUTER_BOUND('',#5888,.T.);
#4840=FACE_OUTER_BOUND('',#5890,.T.);
#4841=FACE_OUTER_BOUND('',#5891,.T.);
#4842=FACE_OUTER_BOUND('',#5892,.T.);
#4843=FACE_OUTER_BOUND('',#5893,.T.);
#4844=FACE_OUTER_BOUND('',#5894,.T.);
#4845=FACE_OUTER_BOUND('',#5895,.T.);
#4846=FACE_OUTER_BOUND('',#5896,.T.);
#4847=FACE_OUTER_BOUND('',#5897,.T.);
#4848=FACE_OUTER_BOUND('',#5898,.T.);
#4849=FACE_OUTER_BOUND('',#5899,.T.);
#4850=FACE_OUTER_BOUND('',#5900,.T.);
#4851=FACE_OUTER_BOUND('',#5901,.T.);
#4852=FACE_OUTER_BOUND('',#5902,.T.);
#4853=FACE_OUTER_BOUND('',#5903,.T.);
#4854=FACE_OUTER_BOUND('',#5905,.T.);
#4855=FACE_OUTER_BOUND('',#5906,.T.);
#4856=FACE_OUTER_BOUND('',#5907,.T.);
#4857=FACE_OUTER_BOUND('',#5908,.T.);
#4858=FACE_OUTER_BOUND('',#5909,.T.);
#4859=FACE_OUTER_BOUND('',#5910,.T.);
#4860=FACE_OUTER_BOUND('',#5911,.T.);
#4861=FACE_OUTER_BOUND('',#5912,.T.);
#4862=FACE_OUTER_BOUND('',#5913,.T.);
#4863=FACE_OUTER_BOUND('',#5914,.T.);
#4864=FACE_OUTER_BOUND('',#5915,.T.);
#4865=FACE_OUTER_BOUND('',#5916,.T.);
#4866=FACE_OUTER_BOUND('',#5917,.T.);
#4867=FACE_OUTER_BOUND('',#5918,.T.);
#4868=FACE_OUTER_BOUND('',#5920,.T.);
#4869=FACE_OUTER_BOUND('',#5921,.T.);
#4870=FACE_OUTER_BOUND('',#5922,.T.);
#4871=FACE_OUTER_BOUND('',#5923,.T.);
#4872=FACE_OUTER_BOUND('',#5924,.T.);
#4873=FACE_OUTER_BOUND('',#5925,.T.);
#4874=FACE_OUTER_BOUND('',#5926,.T.);
#4875=FACE_OUTER_BOUND('',#5927,.T.);
#4876=FACE_OUTER_BOUND('',#5928,.T.);
#4877=FACE_OUTER_BOUND('',#5929,.T.);
#4878=FACE_OUTER_BOUND('',#5930,.T.);
#4879=FACE_OUTER_BOUND('',#5931,.T.);
#4880=FACE_OUTER_BOUND('',#5932,.T.);
#4881=FACE_OUTER_BOUND('',#5933,.T.);
#4882=FACE_OUTER_BOUND('',#5935,.T.);
#4883=FACE_OUTER_BOUND('',#5936,.T.);
#4884=FACE_OUTER_BOUND('',#5937,.T.);
#4885=FACE_OUTER_BOUND('',#5938,.T.);
#4886=FACE_OUTER_BOUND('',#5939,.T.);
#4887=FACE_OUTER_BOUND('',#5940,.T.);
#4888=FACE_OUTER_BOUND('',#5941,.T.);
#4889=FACE_OUTER_BOUND('',#5942,.T.);
#4890=FACE_OUTER_BOUND('',#5943,.T.);
#4891=FACE_OUTER_BOUND('',#5944,.T.);
#4892=FACE_OUTER_BOUND('',#5945,.T.);
#4893=FACE_OUTER_BOUND('',#5946,.T.);
#4894=FACE_OUTER_BOUND('',#5947,.T.);
#4895=FACE_OUTER_BOUND('',#5948,.T.);
#4896=FACE_OUTER_BOUND('',#5950,.T.);
#4897=FACE_OUTER_BOUND('',#5951,.T.);
#4898=FACE_OUTER_BOUND('',#5952,.T.);
#4899=FACE_OUTER_BOUND('',#5953,.T.);
#4900=FACE_OUTER_BOUND('',#5954,.T.);
#4901=FACE_OUTER_BOUND('',#5955,.T.);
#4902=FACE_OUTER_BOUND('',#5956,.T.);
#4903=FACE_OUTER_BOUND('',#5957,.T.);
#4904=FACE_OUTER_BOUND('',#5958,.T.);
#4905=FACE_OUTER_BOUND('',#5959,.T.);
#4906=FACE_OUTER_BOUND('',#5960,.T.);
#4907=FACE_OUTER_BOUND('',#5961,.T.);
#4908=FACE_OUTER_BOUND('',#5962,.T.);
#4909=FACE_OUTER_BOUND('',#5963,.T.);
#4910=FACE_OUTER_BOUND('',#5965,.T.);
#4911=FACE_OUTER_BOUND('',#5966,.T.);
#4912=FACE_OUTER_BOUND('',#5967,.T.);
#4913=FACE_OUTER_BOUND('',#5968,.T.);
#4914=FACE_OUTER_BOUND('',#5969,.T.);
#4915=FACE_OUTER_BOUND('',#5970,.T.);
#4916=FACE_OUTER_BOUND('',#5971,.T.);
#4917=FACE_OUTER_BOUND('',#5972,.T.);
#4918=FACE_OUTER_BOUND('',#5973,.T.);
#4919=FACE_OUTER_BOUND('',#5974,.T.);
#4920=FACE_OUTER_BOUND('',#5975,.T.);
#4921=FACE_OUTER_BOUND('',#5976,.T.);
#4922=FACE_OUTER_BOUND('',#5977,.T.);
#4923=FACE_OUTER_BOUND('',#5978,.T.);
#4924=FACE_OUTER_BOUND('',#5980,.T.);
#4925=FACE_OUTER_BOUND('',#5981,.T.);
#4926=FACE_OUTER_BOUND('',#5982,.T.);
#4927=FACE_OUTER_BOUND('',#5983,.T.);
#4928=FACE_OUTER_BOUND('',#5984,.T.);
#4929=FACE_OUTER_BOUND('',#5985,.T.);
#4930=FACE_OUTER_BOUND('',#5986,.T.);
#4931=FACE_OUTER_BOUND('',#5987,.T.);
#4932=FACE_OUTER_BOUND('',#5988,.T.);
#4933=FACE_OUTER_BOUND('',#5989,.T.);
#4934=FACE_OUTER_BOUND('',#5990,.T.);
#4935=FACE_OUTER_BOUND('',#5991,.T.);
#4936=FACE_OUTER_BOUND('',#5992,.T.);
#4937=FACE_OUTER_BOUND('',#5993,.T.);
#4938=FACE_OUTER_BOUND('',#5995,.T.);
#4939=FACE_OUTER_BOUND('',#5996,.T.);
#4940=FACE_OUTER_BOUND('',#5997,.T.);
#4941=FACE_OUTER_BOUND('',#5998,.T.);
#4942=FACE_OUTER_BOUND('',#5999,.T.);
#4943=FACE_OUTER_BOUND('',#6000,.T.);
#4944=FACE_OUTER_BOUND('',#6001,.T.);
#4945=FACE_OUTER_BOUND('',#6002,.T.);
#4946=FACE_OUTER_BOUND('',#6003,.T.);
#4947=FACE_OUTER_BOUND('',#6004,.T.);
#4948=FACE_OUTER_BOUND('',#6005,.T.);
#4949=FACE_OUTER_BOUND('',#6006,.T.);
#4950=FACE_OUTER_BOUND('',#6007,.T.);
#4951=FACE_OUTER_BOUND('',#6008,.T.);
#4952=FACE_OUTER_BOUND('',#6010,.T.);
#4953=FACE_OUTER_BOUND('',#6011,.T.);
#4954=FACE_OUTER_BOUND('',#6012,.T.);
#4955=FACE_OUTER_BOUND('',#6013,.T.);
#4956=FACE_OUTER_BOUND('',#6014,.T.);
#4957=FACE_OUTER_BOUND('',#6015,.T.);
#4958=FACE_OUTER_BOUND('',#6016,.T.);
#4959=FACE_OUTER_BOUND('',#6017,.T.);
#4960=FACE_OUTER_BOUND('',#6019,.T.);
#4961=FACE_OUTER_BOUND('',#6021,.T.);
#4962=FACE_OUTER_BOUND('',#6023,.T.);
#4963=FACE_OUTER_BOUND('',#6025,.T.);
#4964=FACE_OUTER_BOUND('',#6027,.T.);
#4965=FACE_OUTER_BOUND('',#6029,.T.);
#4966=FACE_OUTER_BOUND('',#6031,.T.);
#4967=FACE_OUTER_BOUND('',#6033,.T.);
#4968=FACE_OUTER_BOUND('',#6034,.T.);
#4969=FACE_OUTER_BOUND('',#6035,.T.);
#4970=FACE_OUTER_BOUND('',#6036,.T.);
#4971=FACE_OUTER_BOUND('',#6037,.T.);
#4972=FACE_OUTER_BOUND('',#6038,.T.);
#4973=FACE_OUTER_BOUND('',#6039,.T.);
#4974=FACE_OUTER_BOUND('',#6040,.T.);
#4975=FACE_OUTER_BOUND('',#6041,.T.);
#4976=FACE_OUTER_BOUND('',#6042,.T.);
#4977=FACE_OUTER_BOUND('',#6043,.T.);
#4978=FACE_OUTER_BOUND('',#6044,.T.);
#4979=FACE_OUTER_BOUND('',#6045,.T.);
#5888=EDGE_LOOP('',(#13046,#13047,#13048,#13049,#13050,#13051,#13052,#13053));
#5889=EDGE_LOOP('',(#13054,#13055,#13056,#13057));
#5890=EDGE_LOOP('',(#13058,#13059,#13060,#13061));
#5891=EDGE_LOOP('',(#13062,#13063,#13064,#13065));
#5892=EDGE_LOOP('',(#13066,#13067,#13068,#13069));
#5893=EDGE_LOOP('',(#13070,#13071,#13072,#13073));
#5894=EDGE_LOOP('',(#13074,#13075,#13076,#13077));
#5895=EDGE_LOOP('',(#13078,#13079,#13080,#13081));
#5896=EDGE_LOOP('',(#13082,#13083,#13084,#13085,#13086,#13087,#13088,#13089));
#5897=EDGE_LOOP('',(#13090,#13091,#13092,#13093));
#5898=EDGE_LOOP('',(#13094,#13095,#13096,#13097));
#5899=EDGE_LOOP('',(#13098,#13099,#13100,#13101));
#5900=EDGE_LOOP('',(#13102,#13103,#13104,#13105));
#5901=EDGE_LOOP('',(#13106,#13107,#13108,#13109));
#5902=EDGE_LOOP('',(#13110,#13111,#13112,#13113));
#5903=EDGE_LOOP('',(#13114,#13115,#13116,#13117,#13118,#13119,#13120,#13121));
#5904=EDGE_LOOP('',(#13122,#13123,#13124,#13125));
#5905=EDGE_LOOP('',(#13126,#13127,#13128,#13129));
#5906=EDGE_LOOP('',(#13130,#13131,#13132,#13133));
#5907=EDGE_LOOP('',(#13134,#13135,#13136,#13137));
#5908=EDGE_LOOP('',(#13138,#13139,#13140,#13141));
#5909=EDGE_LOOP('',(#13142,#13143,#13144,#13145));
#5910=EDGE_LOOP('',(#13146,#13147,#13148,#13149));
#5911=EDGE_LOOP('',(#13150,#13151,#13152,#13153,#13154,#13155,#13156,#13157));
#5912=EDGE_LOOP('',(#13158,#13159,#13160,#13161));
#5913=EDGE_LOOP('',(#13162,#13163,#13164,#13165));
#5914=EDGE_LOOP('',(#13166,#13167,#13168,#13169));
#5915=EDGE_LOOP('',(#13170,#13171,#13172,#13173));
#5916=EDGE_LOOP('',(#13174,#13175,#13176,#13177));
#5917=EDGE_LOOP('',(#13178,#13179,#13180,#13181));
#5918=EDGE_LOOP('',(#13182,#13183,#13184,#13185,#13186,#13187,#13188,#13189));
#5919=EDGE_LOOP('',(#13190,#13191,#13192,#13193));
#5920=EDGE_LOOP('',(#13194,#13195,#13196,#13197));
#5921=EDGE_LOOP('',(#13198,#13199,#13200,#13201));
#5922=EDGE_LOOP('',(#13202,#13203,#13204,#13205));
#5923=EDGE_LOOP('',(#13206,#13207,#13208,#13209));
#5924=EDGE_LOOP('',(#13210,#13211,#13212,#13213));
#5925=EDGE_LOOP('',(#13214,#13215,#13216,#13217));
#5926=EDGE_LOOP('',(#13218,#13219,#13220,#13221,#13222,#13223,#13224,#13225));
#5927=EDGE_LOOP('',(#13226,#13227,#13228,#13229));
#5928=EDGE_LOOP('',(#13230,#13231,#13232,#13233));
#5929=EDGE_LOOP('',(#13234,#13235,#13236,#13237));
#5930=EDGE_LOOP('',(#13238,#13239,#13240,#13241));
#5931=EDGE_LOOP('',(#13242,#13243,#13244,#13245));
#5932=EDGE_LOOP('',(#13246,#13247,#13248,#13249));
#5933=EDGE_LOOP('',(#13250,#13251,#13252,#13253,#13254,#13255,#13256,#13257));
#5934=EDGE_LOOP('',(#13258,#13259,#13260,#13261));
#5935=EDGE_LOOP('',(#13262,#13263,#13264,#13265));
#5936=EDGE_LOOP('',(#13266,#13267,#13268,#13269));
#5937=EDGE_LOOP('',(#13270,#13271,#13272,#13273));
#5938=EDGE_LOOP('',(#13274,#13275,#13276,#13277));
#5939=EDGE_LOOP('',(#13278,#13279,#13280,#13281));
#5940=EDGE_LOOP('',(#13282,#13283,#13284,#13285));
#5941=EDGE_LOOP('',(#13286,#13287,#13288,#13289,#13290,#13291,#13292,#13293));
#5942=EDGE_LOOP('',(#13294,#13295,#13296,#13297));
#5943=EDGE_LOOP('',(#13298,#13299,#13300,#13301));
#5944=EDGE_LOOP('',(#13302,#13303,#13304,#13305));
#5945=EDGE_LOOP('',(#13306,#13307,#13308,#13309));
#5946=EDGE_LOOP('',(#13310,#13311,#13312,#13313));
#5947=EDGE_LOOP('',(#13314,#13315,#13316,#13317));
#5948=EDGE_LOOP('',(#13318,#13319,#13320,#13321,#13322,#13323,#13324,#13325));
#5949=EDGE_LOOP('',(#13326,#13327,#13328,#13329));
#5950=EDGE_LOOP('',(#13330,#13331,#13332,#13333));
#5951=EDGE_LOOP('',(#13334,#13335,#13336,#13337));
#5952=EDGE_LOOP('',(#13338,#13339,#13340,#13341));
#5953=EDGE_LOOP('',(#13342,#13343,#13344,#13345));
#5954=EDGE_LOOP('',(#13346,#13347,#13348,#13349));
#5955=EDGE_LOOP('',(#13350,#13351,#13352,#13353));
#5956=EDGE_LOOP('',(#13354,#13355,#13356,#13357,#13358,#13359,#13360,#13361));
#5957=EDGE_LOOP('',(#13362,#13363,#13364,#13365));
#5958=EDGE_LOOP('',(#13366,#13367,#13368,#13369));
#5959=EDGE_LOOP('',(#13370,#13371,#13372,#13373));
#5960=EDGE_LOOP('',(#13374,#13375,#13376,#13377));
#5961=EDGE_LOOP('',(#13378,#13379,#13380,#13381));
#5962=EDGE_LOOP('',(#13382,#13383,#13384,#13385));
#5963=EDGE_LOOP('',(#13386,#13387,#13388,#13389,#13390,#13391,#13392,#13393));
#5964=EDGE_LOOP('',(#13394,#13395,#13396,#13397));
#5965=EDGE_LOOP('',(#13398,#13399,#13400,#13401));
#5966=EDGE_LOOP('',(#13402,#13403,#13404,#13405));
#5967=EDGE_LOOP('',(#13406,#13407,#13408,#13409));
#5968=EDGE_LOOP('',(#13410,#13411,#13412,#13413));
#5969=EDGE_LOOP('',(#13414,#13415,#13416,#13417));
#5970=EDGE_LOOP('',(#13418,#13419,#13420,#13421));
#5971=EDGE_LOOP('',(#13422,#13423,#13424,#13425,#13426,#13427,#13428,#13429));
#5972=EDGE_LOOP('',(#13430,#13431,#13432,#13433));
#5973=EDGE_LOOP('',(#13434,#13435,#13436,#13437));
#5974=EDGE_LOOP('',(#13438,#13439,#13440,#13441));
#5975=EDGE_LOOP('',(#13442,#13443,#13444,#13445));
#5976=EDGE_LOOP('',(#13446,#13447,#13448,#13449));
#5977=EDGE_LOOP('',(#13450,#13451,#13452,#13453));
#5978=EDGE_LOOP('',(#13454,#13455,#13456,#13457,#13458,#13459,#13460,#13461));
#5979=EDGE_LOOP('',(#13462,#13463,#13464,#13465));
#5980=EDGE_LOOP('',(#13466,#13467,#13468,#13469));
#5981=EDGE_LOOP('',(#13470,#13471,#13472,#13473));
#5982=EDGE_LOOP('',(#13474,#13475,#13476,#13477));
#5983=EDGE_LOOP('',(#13478,#13479,#13480,#13481));
#5984=EDGE_LOOP('',(#13482,#13483,#13484,#13485));
#5985=EDGE_LOOP('',(#13486,#13487,#13488,#13489));
#5986=EDGE_LOOP('',(#13490,#13491,#13492,#13493,#13494,#13495,#13496,#13497));
#5987=EDGE_LOOP('',(#13498,#13499,#13500,#13501));
#5988=EDGE_LOOP('',(#13502,#13503,#13504,#13505));
#5989=EDGE_LOOP('',(#13506,#13507,#13508,#13509));
#5990=EDGE_LOOP('',(#13510,#13511,#13512,#13513));
#5991=EDGE_LOOP('',(#13514,#13515,#13516,#13517));
#5992=EDGE_LOOP('',(#13518,#13519,#13520,#13521));
#5993=EDGE_LOOP('',(#13522,#13523,#13524,#13525,#13526,#13527,#13528,#13529));
#5994=EDGE_LOOP('',(#13530,#13531,#13532,#13533));
#5995=EDGE_LOOP('',(#13534,#13535,#13536,#13537));
#5996=EDGE_LOOP('',(#13538,#13539,#13540,#13541));
#5997=EDGE_LOOP('',(#13542,#13543,#13544,#13545));
#5998=EDGE_LOOP('',(#13546,#13547,#13548,#13549));
#5999=EDGE_LOOP('',(#13550,#13551,#13552,#13553));
#6000=EDGE_LOOP('',(#13554,#13555,#13556,#13557));
#6001=EDGE_LOOP('',(#13558,#13559,#13560,#13561,#13562,#13563,#13564,#13565));
#6002=EDGE_LOOP('',(#13566,#13567,#13568,#13569));
#6003=EDGE_LOOP('',(#13570,#13571,#13572,#13573));
#6004=EDGE_LOOP('',(#13574,#13575,#13576,#13577));
#6005=EDGE_LOOP('',(#13578,#13579,#13580,#13581));
#6006=EDGE_LOOP('',(#13582,#13583,#13584,#13585,#13586,#13587));
#6007=EDGE_LOOP('',(#13588,#13589,#13590,#13591));
#6008=EDGE_LOOP('',(#13592,#13593,#13594,#13595,#13596,#13597,#13598,#13599));
#6009=EDGE_LOOP('',(#13600,#13601,#13602,#13603,#13604,#13605,#13606,#13607));
#6010=EDGE_LOOP('',(#13608,#13609,#13610,#13611));
#6011=EDGE_LOOP('',(#13612,#13613,#13614,#13615));
#6012=EDGE_LOOP('',(#13616,#13617,#13618,#13619,#13620));
#6013=EDGE_LOOP('',(#13621,#13622,#13623,#13624,#13625));
#6014=EDGE_LOOP('',(#13626,#13627,#13628,#13629));
#6015=EDGE_LOOP('',(#13630,#13631,#13632,#13633));
#6016=EDGE_LOOP('',(#13634,#13635,#13636,#13637));
#6017=EDGE_LOOP('',(#13638,#13639,#13640,#13641,#13642,#13643,#13644,#13645,
#13646,#13647));
#6018=EDGE_LOOP('',(#13648,#13649,#13650,#13651,#13652,#13653,#13654,#13655,
#13656,#13657,#13658,#13659));
#6019=EDGE_LOOP('',(#13660,#13661,#13662,#13663));
#6020=EDGE_LOOP('',(#13664,#13665,#13666,#13667));
#6021=EDGE_LOOP('',(#13668,#13669,#13670,#13671));
#6022=EDGE_LOOP('',(#13672,#13673,#13674,#13675));
#6023=EDGE_LOOP('',(#13676,#13677,#13678,#13679));
#6024=EDGE_LOOP('',(#13680,#13681,#13682,#13683));
#6025=EDGE_LOOP('',(#13684,#13685,#13686,#13687));
#6026=EDGE_LOOP('',(#13688,#13689,#13690,#13691));
#6027=EDGE_LOOP('',(#13692,#13693,#13694,#13695));
#6028=EDGE_LOOP('',(#13696,#13697,#13698,#13699));
#6029=EDGE_LOOP('',(#13700,#13701,#13702,#13703));
#6030=EDGE_LOOP('',(#13704,#13705,#13706,#13707));
#6031=EDGE_LOOP('',(#13708,#13709,#13710,#13711));
#6032=EDGE_LOOP('',(#13712,#13713,#13714,#13715));
#6033=EDGE_LOOP('',(#13716,#13717,#13718,#13719,#13720,#13721));
#6034=EDGE_LOOP('',(#13722,#13723,#13724,#13725,#13726,#13727,#13728));
#6035=EDGE_LOOP('',(#13729,#13730,#13731,#13732,#13733,#13734,#13735));
#6036=EDGE_LOOP('',(#13736,#13737));
#6037=EDGE_LOOP('',(#13738,#13739,#13740,#13741,#13742,#13743,#13744,#13745));
#6038=EDGE_LOOP('',(#13746,#13747,#13748,#13749));
#6039=EDGE_LOOP('',(#13750,#13751,#13752,#13753));
#6040=EDGE_LOOP('',(#13754,#13755,#13756,#13757));
#6041=EDGE_LOOP('',(#13758,#13759,#13760,#13761));
#6042=EDGE_LOOP('',(#13762,#13763,#13764,#13765,#13766,#13767,#13768,#13769,
#13770,#13771,#13772,#13773,#13774,#13775));
#6043=EDGE_LOOP('',(#13776,#13777,#13778,#13779,#13780,#13781));
#6044=EDGE_LOOP('',(#13782,#13783,#13784,#13785));
#6045=EDGE_LOOP('',(#13786,#13787,#13788,#13789));
#7051=CIRCLE('',#20062,0.01465000000001);
#7052=CIRCLE('',#20065,0.01465000000001);
#7053=CIRCLE('',#20071,0.01390000000001);
#7054=CIRCLE('',#20079,0.01390000000001);
#7055=CIRCLE('',#20084,0.00150000000001414);
#7056=CIRCLE('',#20086,0.00150000000001414);
#7057=CIRCLE('',#20090,0.0146500000000141);
#7058=CIRCLE('',#20093,0.0146500000000141);
#7059=CIRCLE('',#20099,0.0139000000000141);
#7060=CIRCLE('',#20107,0.0139000000000141);
#7061=CIRCLE('',#20112,0.00150000000001);
#7062=CIRCLE('',#20114,0.00150000000001);
#7063=CIRCLE('',#20118,0.01465000000001);
#7064=CIRCLE('',#20121,0.01465000000001);
#7065=CIRCLE('',#20127,0.01390000000001);
#7066=CIRCLE('',#20135,0.01390000000001);
#7067=CIRCLE('',#20140,0.00150000000001414);
#7068=CIRCLE('',#20142,0.00150000000001414);
#7069=CIRCLE('',#20146,0.0146500000000141);
#7070=CIRCLE('',#20149,0.0146500000000141);
#7071=CIRCLE('',#20155,0.0139000000000141);
#7072=CIRCLE('',#20163,0.0139000000000141);
#7073=CIRCLE('',#20168,0.00150000000001);
#7074=CIRCLE('',#20170,0.00150000000001);
#7075=CIRCLE('',#20174,0.01465000000001);
#7076=CIRCLE('',#20177,0.01465000000001);
#7077=CIRCLE('',#20183,0.01390000000001);
#7078=CIRCLE('',#20191,0.01390000000001);
#7079=CIRCLE('',#20196,0.00150000000001414);
#7080=CIRCLE('',#20198,0.00150000000001414);
#7081=CIRCLE('',#20202,0.0146500000000141);
#7082=CIRCLE('',#20205,0.0146500000000141);
#7083=CIRCLE('',#20211,0.0139000000000141);
#7084=CIRCLE('',#20219,0.0139000000000141);
#7085=CIRCLE('',#20224,0.00150000000001);
#7086=CIRCLE('',#20226,0.00150000000001);
#7087=CIRCLE('',#20230,0.01465000000001);
#7088=CIRCLE('',#20233,0.01465000000001);
#7089=CIRCLE('',#20239,0.01390000000001);
#7090=CIRCLE('',#20247,0.01390000000001);
#7091=CIRCLE('',#20252,0.00150000000001414);
#7092=CIRCLE('',#20254,0.00150000000001414);
#7093=CIRCLE('',#20258,0.0146500000000141);
#7094=CIRCLE('',#20261,0.0146500000000141);
#7095=CIRCLE('',#20267,0.0139000000000141);
#7096=CIRCLE('',#20275,0.0139000000000141);
#7097=CIRCLE('',#20280,0.00150000000001);
#7098=CIRCLE('',#20282,0.00150000000001);
#7099=CIRCLE('',#20283,0.00150000000001);
#7100=CIRCLE('',#20284,0.00150000000001);
#8153=VERTEX_POINT('',#28723);
#8154=VERTEX_POINT('',#28724);
#8155=VERTEX_POINT('',#28726);
#8156=VERTEX_POINT('',#28728);
#8157=VERTEX_POINT('',#28730);
#8158=VERTEX_POINT('',#28732);
#8159=VERTEX_POINT('',#28734);
#8160=VERTEX_POINT('',#28736);
#8161=VERTEX_POINT('',#28739);
#8162=VERTEX_POINT('',#28740);
#8163=VERTEX_POINT('',#28742);
#8164=VERTEX_POINT('',#28761);
#8165=VERTEX_POINT('',#28782);
#8166=VERTEX_POINT('',#28784);
#8167=VERTEX_POINT('',#28788);
#8168=VERTEX_POINT('',#28792);
#8169=VERTEX_POINT('',#28796);
#8170=VERTEX_POINT('',#28800);
#8171=VERTEX_POINT('',#28804);
#8172=VERTEX_POINT('',#28808);
#8173=VERTEX_POINT('',#28815);
#8174=VERTEX_POINT('',#28817);
#8175=VERTEX_POINT('',#28821);
#8176=VERTEX_POINT('',#28825);
#8177=VERTEX_POINT('',#28831);
#8178=VERTEX_POINT('',#28832);
#8179=VERTEX_POINT('',#28834);
#8180=VERTEX_POINT('',#28836);
#8181=VERTEX_POINT('',#28838);
#8182=VERTEX_POINT('',#28840);
#8183=VERTEX_POINT('',#28842);
#8184=VERTEX_POINT('',#28844);
#8185=VERTEX_POINT('',#28847);
#8186=VERTEX_POINT('',#28848);
#8187=VERTEX_POINT('',#28850);
#8188=VERTEX_POINT('',#28869);
#8189=VERTEX_POINT('',#28890);
#8190=VERTEX_POINT('',#28892);
#8191=VERTEX_POINT('',#28896);
#8192=VERTEX_POINT('',#28900);
#8193=VERTEX_POINT('',#28904);
#8194=VERTEX_POINT('',#28908);
#8195=VERTEX_POINT('',#28912);
#8196=VERTEX_POINT('',#28916);
#8197=VERTEX_POINT('',#28923);
#8198=VERTEX_POINT('',#28925);
#8199=VERTEX_POINT('',#28929);
#8200=VERTEX_POINT('',#28933);
#8201=VERTEX_POINT('',#28939);
#8202=VERTEX_POINT('',#28940);
#8203=VERTEX_POINT('',#28942);
#8204=VERTEX_POINT('',#28944);
#8205=VERTEX_POINT('',#28946);
#8206=VERTEX_POINT('',#28948);
#8207=VERTEX_POINT('',#28950);
#8208=VERTEX_POINT('',#28952);
#8209=VERTEX_POINT('',#28955);
#8210=VERTEX_POINT('',#28956);
#8211=VERTEX_POINT('',#28958);
#8212=VERTEX_POINT('',#28977);
#8213=VERTEX_POINT('',#28998);
#8214=VERTEX_POINT('',#29000);
#8215=VERTEX_POINT('',#29004);
#8216=VERTEX_POINT('',#29008);
#8217=VERTEX_POINT('',#29012);
#8218=VERTEX_POINT('',#29016);
#8219=VERTEX_POINT('',#29020);
#8220=VERTEX_POINT('',#29024);
#8221=VERTEX_POINT('',#29031);
#8222=VERTEX_POINT('',#29033);
#8223=VERTEX_POINT('',#29037);
#8224=VERTEX_POINT('',#29041);
#8225=VERTEX_POINT('',#29047);
#8226=VERTEX_POINT('',#29048);
#8227=VERTEX_POINT('',#29050);
#8228=VERTEX_POINT('',#29052);
#8229=VERTEX_POINT('',#29054);
#8230=VERTEX_POINT('',#29056);
#8231=VERTEX_POINT('',#29058);
#8232=VERTEX_POINT('',#29060);
#8233=VERTEX_POINT('',#29063);
#8234=VERTEX_POINT('',#29064);
#8235=VERTEX_POINT('',#29066);
#8236=VERTEX_POINT('',#29085);
#8237=VERTEX_POINT('',#29106);
#8238=VERTEX_POINT('',#29108);
#8239=VERTEX_POINT('',#29112);
#8240=VERTEX_POINT('',#29116);
#8241=VERTEX_POINT('',#29120);
#8242=VERTEX_POINT('',#29124);
#8243=VERTEX_POINT('',#29128);
#8244=VERTEX_POINT('',#29132);
#8245=VERTEX_POINT('',#29139);
#8246=VERTEX_POINT('',#29141);
#8247=VERTEX_POINT('',#29145);
#8248=VERTEX_POINT('',#29149);
#8249=VERTEX_POINT('',#29155);
#8250=VERTEX_POINT('',#29156);
#8251=VERTEX_POINT('',#29158);
#8252=VERTEX_POINT('',#29160);
#8253=VERTEX_POINT('',#29162);
#8254=VERTEX_POINT('',#29164);
#8255=VERTEX_POINT('',#29166);
#8256=VERTEX_POINT('',#29168);
#8257=VERTEX_POINT('',#29171);
#8258=VERTEX_POINT('',#29172);
#8259=VERTEX_POINT('',#29174);
#8260=VERTEX_POINT('',#29193);
#8261=VERTEX_POINT('',#29214);
#8262=VERTEX_POINT('',#29216);
#8263=VERTEX_POINT('',#29220);
#8264=VERTEX_POINT('',#29224);
#8265=VERTEX_POINT('',#29228);
#8266=VERTEX_POINT('',#29232);
#8267=VERTEX_POINT('',#29236);
#8268=VERTEX_POINT('',#29240);
#8269=VERTEX_POINT('',#29247);
#8270=VERTEX_POINT('',#29249);
#8271=VERTEX_POINT('',#29253);
#8272=VERTEX_POINT('',#29257);
#8273=VERTEX_POINT('',#29263);
#8274=VERTEX_POINT('',#29264);
#8275=VERTEX_POINT('',#29266);
#8276=VERTEX_POINT('',#29268);
#8277=VERTEX_POINT('',#29270);
#8278=VERTEX_POINT('',#29272);
#8279=VERTEX_POINT('',#29274);
#8280=VERTEX_POINT('',#29276);
#8281=VERTEX_POINT('',#29279);
#8282=VERTEX_POINT('',#29280);
#8283=VERTEX_POINT('',#29282);
#8284=VERTEX_POINT('',#29301);
#8285=VERTEX_POINT('',#29322);
#8286=VERTEX_POINT('',#29324);
#8287=VERTEX_POINT('',#29328);
#8288=VERTEX_POINT('',#29332);
#8289=VERTEX_POINT('',#29336);
#8290=VERTEX_POINT('',#29340);
#8291=VERTEX_POINT('',#29344);
#8292=VERTEX_POINT('',#29348);
#8293=VERTEX_POINT('',#29355);
#8294=VERTEX_POINT('',#29357);
#8295=VERTEX_POINT('',#29361);
#8296=VERTEX_POINT('',#29365);
#8297=VERTEX_POINT('',#29371);
#8298=VERTEX_POINT('',#29372);
#8299=VERTEX_POINT('',#29374);
#8300=VERTEX_POINT('',#29376);
#8301=VERTEX_POINT('',#29378);
#8302=VERTEX_POINT('',#29380);
#8303=VERTEX_POINT('',#29382);
#8304=VERTEX_POINT('',#29384);
#8305=VERTEX_POINT('',#29387);
#8306=VERTEX_POINT('',#29388);
#8307=VERTEX_POINT('',#29390);
#8308=VERTEX_POINT('',#29409);
#8309=VERTEX_POINT('',#29430);
#8310=VERTEX_POINT('',#29432);
#8311=VERTEX_POINT('',#29436);
#8312=VERTEX_POINT('',#29440);
#8313=VERTEX_POINT('',#29444);
#8314=VERTEX_POINT('',#29448);
#8315=VERTEX_POINT('',#29452);
#8316=VERTEX_POINT('',#29456);
#8317=VERTEX_POINT('',#29463);
#8318=VERTEX_POINT('',#29465);
#8319=VERTEX_POINT('',#29469);
#8320=VERTEX_POINT('',#29473);
#8321=VERTEX_POINT('',#29479);
#8322=VERTEX_POINT('',#29480);
#8323=VERTEX_POINT('',#29482);
#8324=VERTEX_POINT('',#29484);
#8325=VERTEX_POINT('',#29486);
#8326=VERTEX_POINT('',#29488);
#8327=VERTEX_POINT('',#29490);
#8328=VERTEX_POINT('',#29492);
#8329=VERTEX_POINT('',#29495);
#8330=VERTEX_POINT('',#29496);
#8331=VERTEX_POINT('',#29498);
#8332=VERTEX_POINT('',#29517);
#8333=VERTEX_POINT('',#29538);
#8334=VERTEX_POINT('',#29540);
#8335=VERTEX_POINT('',#29544);
#8336=VERTEX_POINT('',#29548);
#8337=VERTEX_POINT('',#29552);
#8338=VERTEX_POINT('',#29556);
#8339=VERTEX_POINT('',#29560);
#8340=VERTEX_POINT('',#29564);
#8341=VERTEX_POINT('',#29571);
#8342=VERTEX_POINT('',#29573);
#8343=VERTEX_POINT('',#29577);
#8344=VERTEX_POINT('',#29581);
#8345=VERTEX_POINT('',#29583);
#8346=VERTEX_POINT('',#29585);
#8347=VERTEX_POINT('',#29591);
#8348=VERTEX_POINT('',#29592);
#8349=VERTEX_POINT('',#29594);
#8350=VERTEX_POINT('',#29596);
#8351=VERTEX_POINT('',#29598);
#8352=VERTEX_POINT('',#29600);
#8353=VERTEX_POINT('',#29602);
#8354=VERTEX_POINT('',#29604);
#8355=VERTEX_POINT('',#29607);
#8356=VERTEX_POINT('',#29608);
#8357=VERTEX_POINT('',#29610);
#8358=VERTEX_POINT('',#29612);
#8359=VERTEX_POINT('',#29614);
#8360=VERTEX_POINT('',#29616);
#8361=VERTEX_POINT('',#29618);
#8362=VERTEX_POINT('',#29620);
#8363=VERTEX_POINT('',#29624);
#8364=VERTEX_POINT('',#29626);
#8365=VERTEX_POINT('',#29630);
#8366=VERTEX_POINT('',#29634);
#8367=VERTEX_POINT('',#29635);
#8368=VERTEX_POINT('',#29640);
#8369=VERTEX_POINT('',#29642);
#8370=VERTEX_POINT('',#29644);
#8371=VERTEX_POINT('',#29648);
#8372=VERTEX_POINT('',#29652);
#8373=VERTEX_POINT('',#29658);
#8374=VERTEX_POINT('',#29660);
#8375=VERTEX_POINT('',#29663);
#8376=VERTEX_POINT('',#29664);
#8377=VERTEX_POINT('',#29666);
#8378=VERTEX_POINT('',#29668);
#8379=VERTEX_POINT('',#29670);
#8380=VERTEX_POINT('',#29672);
#8381=VERTEX_POINT('',#29674);
#8382=VERTEX_POINT('',#29676);
#8383=VERTEX_POINT('',#29678);
#8384=VERTEX_POINT('',#29680);
#8385=VERTEX_POINT('',#29682);
#8386=VERTEX_POINT('',#29684);
#8387=VERTEX_POINT('',#29703);
#8388=VERTEX_POINT('',#29705);
#8389=VERTEX_POINT('',#29707);
#8390=VERTEX_POINT('',#29709);
#8391=VERTEX_POINT('',#29714);
#8392=VERTEX_POINT('',#29715);
#8393=VERTEX_POINT('',#29717);
#8394=VERTEX_POINT('',#29723);
#8395=VERTEX_POINT('',#29725);
#8396=VERTEX_POINT('',#29727);
#8397=VERTEX_POINT('',#29733);
#8398=VERTEX_POINT('',#29736);
#10081=EDGE_CURVE('',#8153,#8154,#236,.T.);
#10082=EDGE_CURVE('',#8153,#8155,#7051,.T.);
#10083=EDGE_CURVE('',#8156,#8155,#237,.T.);
#10084=EDGE_CURVE('',#8156,#8157,#1145,.T.);
#10085=EDGE_CURVE('',#8158,#8157,#238,.T.);
#10086=EDGE_CURVE('',#8159,#8158,#7052,.T.);
#10087=EDGE_CURVE('',#8160,#8159,#239,.T.);
#10088=EDGE_CURVE('',#8160,#8154,#1146,.T.);
#10089=EDGE_CURVE('',#8161,#8162,#1147,.T.);
#10090=EDGE_CURVE('',#8162,#8163,#200,.T.);
#10091=EDGE_CURVE('',#8163,#8164,#1148,.T.);
#10092=EDGE_CURVE('',#8164,#8161,#201,.T.);
#10093=EDGE_CURVE('',#8154,#8165,#1149,.T.);
#10094=EDGE_CURVE('',#8166,#8160,#1150,.T.);
#10095=EDGE_CURVE('',#8165,#8166,#1151,.T.);
#10096=EDGE_CURVE('',#8159,#8167,#1152,.T.);
#10097=EDGE_CURVE('',#8167,#8166,#240,.T.);
#10098=EDGE_CURVE('',#8168,#8158,#1153,.T.);
#10099=EDGE_CURVE('',#8168,#8167,#7053,.T.);
#10100=EDGE_CURVE('',#8169,#8168,#241,.T.);
#10101=EDGE_CURVE('',#8157,#8169,#1154,.T.);
#10102=EDGE_CURVE('',#8170,#8156,#1155,.T.);
#10103=EDGE_CURVE('',#8169,#8170,#1156,.T.);
#10104=EDGE_CURVE('',#8155,#8171,#1157,.T.);
#10105=EDGE_CURVE('',#8171,#8170,#242,.T.);
#10106=EDGE_CURVE('',#8165,#8172,#243,.T.);
#10107=EDGE_CURVE('',#8171,#8172,#7054,.T.);
#10108=EDGE_CURVE('',#8172,#8153,#1158,.T.);
#10109=EDGE_CURVE('',#8173,#8163,#1159,.T.);
#10110=EDGE_CURVE('',#8173,#8174,#1160,.T.);
#10111=EDGE_CURVE('',#8174,#8164,#1161,.T.);
#10112=EDGE_CURVE('',#8175,#8162,#1162,.T.);
#10113=EDGE_CURVE('',#8175,#8173,#7055,.T.);
#10114=EDGE_CURVE('',#8174,#8176,#7056,.T.);
#10115=EDGE_CURVE('',#8176,#8161,#1163,.T.);
#10116=EDGE_CURVE('',#8176,#8175,#1164,.T.);
#10117=EDGE_CURVE('',#8177,#8178,#244,.T.);
#10118=EDGE_CURVE('',#8177,#8179,#7057,.T.);
#10119=EDGE_CURVE('',#8180,#8179,#245,.T.);
#10120=EDGE_CURVE('',#8180,#8181,#1165,.T.);
#10121=EDGE_CURVE('',#8182,#8181,#246,.T.);
#10122=EDGE_CURVE('',#8183,#8182,#7058,.T.);
#10123=EDGE_CURVE('',#8184,#8183,#247,.T.);
#10124=EDGE_CURVE('',#8184,#8178,#1166,.T.);
#10125=EDGE_CURVE('',#8185,#8186,#1167,.T.);
#10126=EDGE_CURVE('',#8186,#8187,#202,.T.);
#10127=EDGE_CURVE('',#8187,#8188,#1168,.T.);
#10128=EDGE_CURVE('',#8188,#8185,#203,.T.);
#10129=EDGE_CURVE('',#8178,#8189,#1169,.T.);
#10130=EDGE_CURVE('',#8190,#8184,#1170,.T.);
#10131=EDGE_CURVE('',#8189,#8190,#1171,.T.);
#10132=EDGE_CURVE('',#8183,#8191,#1172,.T.);
#10133=EDGE_CURVE('',#8191,#8190,#248,.T.);
#10134=EDGE_CURVE('',#8192,#8182,#1173,.T.);
#10135=EDGE_CURVE('',#8192,#8191,#7059,.T.);
#10136=EDGE_CURVE('',#8193,#8192,#249,.T.);
#10137=EDGE_CURVE('',#8181,#8193,#1174,.T.);
#10138=EDGE_CURVE('',#8194,#8180,#1175,.T.);
#10139=EDGE_CURVE('',#8193,#8194,#1176,.T.);
#10140=EDGE_CURVE('',#8179,#8195,#1177,.T.);
#10141=EDGE_CURVE('',#8195,#8194,#250,.T.);
#10142=EDGE_CURVE('',#8189,#8196,#251,.T.);
#10143=EDGE_CURVE('',#8195,#8196,#7060,.T.);
#10144=EDGE_CURVE('',#8196,#8177,#1178,.T.);
#10145=EDGE_CURVE('',#8197,#8187,#1179,.T.);
#10146=EDGE_CURVE('',#8197,#8198,#1180,.T.);
#10147=EDGE_CURVE('',#8198,#8188,#1181,.T.);
#10148=EDGE_CURVE('',#8199,#8186,#1182,.T.);
#10149=EDGE_CURVE('',#8199,#8197,#7061,.T.);
#10150=EDGE_CURVE('',#8198,#8200,#7062,.T.);
#10151=EDGE_CURVE('',#8200,#8185,#1183,.T.);
#10152=EDGE_CURVE('',#8200,#8199,#1184,.T.);
#10153=EDGE_CURVE('',#8201,#8202,#252,.T.);
#10154=EDGE_CURVE('',#8201,#8203,#7063,.T.);
#10155=EDGE_CURVE('',#8204,#8203,#253,.T.);
#10156=EDGE_CURVE('',#8204,#8205,#1185,.T.);
#10157=EDGE_CURVE('',#8206,#8205,#254,.T.);
#10158=EDGE_CURVE('',#8207,#8206,#7064,.T.);
#10159=EDGE_CURVE('',#8208,#8207,#255,.T.);
#10160=EDGE_CURVE('',#8208,#8202,#1186,.T.);
#10161=EDGE_CURVE('',#8209,#8210,#1187,.T.);
#10162=EDGE_CURVE('',#8210,#8211,#204,.T.);
#10163=EDGE_CURVE('',#8211,#8212,#1188,.T.);
#10164=EDGE_CURVE('',#8212,#8209,#205,.T.);
#10165=EDGE_CURVE('',#8202,#8213,#1189,.T.);
#10166=EDGE_CURVE('',#8214,#8208,#1190,.T.);
#10167=EDGE_CURVE('',#8213,#8214,#1191,.T.);
#10168=EDGE_CURVE('',#8207,#8215,#1192,.T.);
#10169=EDGE_CURVE('',#8215,#8214,#256,.T.);
#10170=EDGE_CURVE('',#8216,#8206,#1193,.T.);
#10171=EDGE_CURVE('',#8216,#8215,#7065,.T.);
#10172=EDGE_CURVE('',#8217,#8216,#257,.T.);
#10173=EDGE_CURVE('',#8205,#8217,#1194,.T.);
#10174=EDGE_CURVE('',#8218,#8204,#1195,.T.);
#10175=EDGE_CURVE('',#8217,#8218,#1196,.T.);
#10176=EDGE_CURVE('',#8203,#8219,#1197,.T.);
#10177=EDGE_CURVE('',#8219,#8218,#258,.T.);
#10178=EDGE_CURVE('',#8213,#8220,#259,.T.);
#10179=EDGE_CURVE('',#8219,#8220,#7066,.T.);
#10180=EDGE_CURVE('',#8220,#8201,#1198,.T.);
#10181=EDGE_CURVE('',#8221,#8211,#1199,.T.);
#10182=EDGE_CURVE('',#8221,#8222,#1200,.T.);
#10183=EDGE_CURVE('',#8222,#8212,#1201,.T.);
#10184=EDGE_CURVE('',#8223,#8210,#1202,.T.);
#10185=EDGE_CURVE('',#8223,#8221,#7067,.T.);
#10186=EDGE_CURVE('',#8222,#8224,#7068,.T.);
#10187=EDGE_CURVE('',#8224,#8209,#1203,.T.);
#10188=EDGE_CURVE('',#8224,#8223,#1204,.T.);
#10189=EDGE_CURVE('',#8225,#8226,#260,.T.);
#10190=EDGE_CURVE('',#8225,#8227,#7069,.T.);
#10191=EDGE_CURVE('',#8228,#8227,#261,.T.);
#10192=EDGE_CURVE('',#8228,#8229,#1205,.T.);
#10193=EDGE_CURVE('',#8230,#8229,#262,.T.);
#10194=EDGE_CURVE('',#8231,#8230,#7070,.T.);
#10195=EDGE_CURVE('',#8232,#8231,#263,.T.);
#10196=EDGE_CURVE('',#8232,#8226,#1206,.T.);
#10197=EDGE_CURVE('',#8233,#8234,#1207,.T.);
#10198=EDGE_CURVE('',#8234,#8235,#206,.T.);
#10199=EDGE_CURVE('',#8235,#8236,#1208,.T.);
#10200=EDGE_CURVE('',#8236,#8233,#207,.T.);
#10201=EDGE_CURVE('',#8226,#8237,#1209,.T.);
#10202=EDGE_CURVE('',#8238,#8232,#1210,.T.);
#10203=EDGE_CURVE('',#8237,#8238,#1211,.T.);
#10204=EDGE_CURVE('',#8231,#8239,#1212,.T.);
#10205=EDGE_CURVE('',#8239,#8238,#264,.T.);
#10206=EDGE_CURVE('',#8240,#8230,#1213,.T.);
#10207=EDGE_CURVE('',#8240,#8239,#7071,.T.);
#10208=EDGE_CURVE('',#8241,#8240,#265,.T.);
#10209=EDGE_CURVE('',#8229,#8241,#1214,.T.);
#10210=EDGE_CURVE('',#8242,#8228,#1215,.T.);
#10211=EDGE_CURVE('',#8241,#8242,#1216,.T.);
#10212=EDGE_CURVE('',#8227,#8243,#1217,.T.);
#10213=EDGE_CURVE('',#8243,#8242,#266,.T.);
#10214=EDGE_CURVE('',#8237,#8244,#267,.T.);
#10215=EDGE_CURVE('',#8243,#8244,#7072,.T.);
#10216=EDGE_CURVE('',#8244,#8225,#1218,.T.);
#10217=EDGE_CURVE('',#8245,#8235,#1219,.T.);
#10218=EDGE_CURVE('',#8245,#8246,#1220,.T.);
#10219=EDGE_CURVE('',#8246,#8236,#1221,.T.);
#10220=EDGE_CURVE('',#8247,#8234,#1222,.T.);
#10221=EDGE_CURVE('',#8247,#8245,#7073,.T.);
#10222=EDGE_CURVE('',#8246,#8248,#7074,.T.);
#10223=EDGE_CURVE('',#8248,#8233,#1223,.T.);
#10224=EDGE_CURVE('',#8248,#8247,#1224,.T.);
#10225=EDGE_CURVE('',#8249,#8250,#268,.T.);
#10226=EDGE_CURVE('',#8249,#8251,#7075,.T.);
#10227=EDGE_CURVE('',#8252,#8251,#269,.T.);
#10228=EDGE_CURVE('',#8252,#8253,#1225,.T.);
#10229=EDGE_CURVE('',#8254,#8253,#270,.T.);
#10230=EDGE_CURVE('',#8255,#8254,#7076,.T.);
#10231=EDGE_CURVE('',#8256,#8255,#271,.T.);
#10232=EDGE_CURVE('',#8256,#8250,#1226,.T.);
#10233=EDGE_CURVE('',#8257,#8258,#1227,.T.);
#10234=EDGE_CURVE('',#8258,#8259,#208,.T.);
#10235=EDGE_CURVE('',#8259,#8260,#1228,.T.);
#10236=EDGE_CURVE('',#8260,#8257,#209,.T.);
#10237=EDGE_CURVE('',#8250,#8261,#1229,.T.);
#10238=EDGE_CURVE('',#8262,#8256,#1230,.T.);
#10239=EDGE_CURVE('',#8261,#8262,#1231,.T.);
#10240=EDGE_CURVE('',#8255,#8263,#1232,.T.);
#10241=EDGE_CURVE('',#8263,#8262,#272,.T.);
#10242=EDGE_CURVE('',#8264,#8254,#1233,.T.);
#10243=EDGE_CURVE('',#8264,#8263,#7077,.T.);
#10244=EDGE_CURVE('',#8265,#8264,#273,.T.);
#10245=EDGE_CURVE('',#8253,#8265,#1234,.T.);
#10246=EDGE_CURVE('',#8266,#8252,#1235,.T.);
#10247=EDGE_CURVE('',#8265,#8266,#1236,.T.);
#10248=EDGE_CURVE('',#8251,#8267,#1237,.T.);
#10249=EDGE_CURVE('',#8267,#8266,#274,.T.);
#10250=EDGE_CURVE('',#8261,#8268,#275,.T.);
#10251=EDGE_CURVE('',#8267,#8268,#7078,.T.);
#10252=EDGE_CURVE('',#8268,#8249,#1238,.T.);
#10253=EDGE_CURVE('',#8269,#8259,#1239,.T.);
#10254=EDGE_CURVE('',#8269,#8270,#1240,.T.);
#10255=EDGE_CURVE('',#8270,#8260,#1241,.T.);
#10256=EDGE_CURVE('',#8271,#8258,#1242,.T.);
#10257=EDGE_CURVE('',#8271,#8269,#7079,.T.);
#10258=EDGE_CURVE('',#8270,#8272,#7080,.T.);
#10259=EDGE_CURVE('',#8272,#8257,#1243,.T.);
#10260=EDGE_CURVE('',#8272,#8271,#1244,.T.);
#10261=EDGE_CURVE('',#8273,#8274,#276,.T.);
#10262=EDGE_CURVE('',#8273,#8275,#7081,.T.);
#10263=EDGE_CURVE('',#8276,#8275,#277,.T.);
#10264=EDGE_CURVE('',#8276,#8277,#1245,.T.);
#10265=EDGE_CURVE('',#8278,#8277,#278,.T.);
#10266=EDGE_CURVE('',#8279,#8278,#7082,.T.);
#10267=EDGE_CURVE('',#8280,#8279,#279,.T.);
#10268=EDGE_CURVE('',#8280,#8274,#1246,.T.);
#10269=EDGE_CURVE('',#8281,#8282,#1247,.T.);
#10270=EDGE_CURVE('',#8282,#8283,#210,.T.);
#10271=EDGE_CURVE('',#8283,#8284,#1248,.T.);
#10272=EDGE_CURVE('',#8284,#8281,#211,.T.);
#10273=EDGE_CURVE('',#8274,#8285,#1249,.T.);
#10274=EDGE_CURVE('',#8286,#8280,#1250,.T.);
#10275=EDGE_CURVE('',#8285,#8286,#1251,.T.);
#10276=EDGE_CURVE('',#8279,#8287,#1252,.T.);
#10277=EDGE_CURVE('',#8287,#8286,#280,.T.);
#10278=EDGE_CURVE('',#8288,#8278,#1253,.T.);
#10279=EDGE_CURVE('',#8288,#8287,#7083,.T.);
#10280=EDGE_CURVE('',#8289,#8288,#281,.T.);
#10281=EDGE_CURVE('',#8277,#8289,#1254,.T.);
#10282=EDGE_CURVE('',#8290,#8276,#1255,.T.);
#10283=EDGE_CURVE('',#8289,#8290,#1256,.T.);
#10284=EDGE_CURVE('',#8275,#8291,#1257,.T.);
#10285=EDGE_CURVE('',#8291,#8290,#282,.T.);
#10286=EDGE_CURVE('',#8285,#8292,#283,.T.);
#10287=EDGE_CURVE('',#8291,#8292,#7084,.T.);
#10288=EDGE_CURVE('',#8292,#8273,#1258,.T.);
#10289=EDGE_CURVE('',#8293,#8283,#1259,.T.);
#10290=EDGE_CURVE('',#8293,#8294,#1260,.T.);
#10291=EDGE_CURVE('',#8294,#8284,#1261,.T.);
#10292=EDGE_CURVE('',#8295,#8282,#1262,.T.);
#10293=EDGE_CURVE('',#8295,#8293,#7085,.T.);
#10294=EDGE_CURVE('',#8294,#8296,#7086,.T.);
#10295=EDGE_CURVE('',#8296,#8281,#1263,.T.);
#10296=EDGE_CURVE('',#8296,#8295,#1264,.T.);
#10297=EDGE_CURVE('',#8297,#8298,#284,.T.);
#10298=EDGE_CURVE('',#8297,#8299,#7087,.T.);
#10299=EDGE_CURVE('',#8300,#8299,#285,.T.);
#10300=EDGE_CURVE('',#8300,#8301,#1265,.T.);
#10301=EDGE_CURVE('',#8302,#8301,#286,.T.);
#10302=EDGE_CURVE('',#8303,#8302,#7088,.T.);
#10303=EDGE_CURVE('',#8304,#8303,#287,.T.);
#10304=EDGE_CURVE('',#8304,#8298,#1266,.T.);
#10305=EDGE_CURVE('',#8305,#8306,#1267,.T.);
#10306=EDGE_CURVE('',#8306,#8307,#212,.T.);
#10307=EDGE_CURVE('',#8307,#8308,#1268,.T.);
#10308=EDGE_CURVE('',#8308,#8305,#213,.T.);
#10309=EDGE_CURVE('',#8298,#8309,#1269,.T.);
#10310=EDGE_CURVE('',#8310,#8304,#1270,.T.);
#10311=EDGE_CURVE('',#8309,#8310,#1271,.T.);
#10312=EDGE_CURVE('',#8303,#8311,#1272,.T.);
#10313=EDGE_CURVE('',#8311,#8310,#288,.T.);
#10314=EDGE_CURVE('',#8312,#8302,#1273,.T.);
#10315=EDGE_CURVE('',#8312,#8311,#7089,.T.);
#10316=EDGE_CURVE('',#8313,#8312,#289,.T.);
#10317=EDGE_CURVE('',#8301,#8313,#1274,.T.);
#10318=EDGE_CURVE('',#8314,#8300,#1275,.T.);
#10319=EDGE_CURVE('',#8313,#8314,#1276,.T.);
#10320=EDGE_CURVE('',#8299,#8315,#1277,.T.);
#10321=EDGE_CURVE('',#8315,#8314,#290,.T.);
#10322=EDGE_CURVE('',#8309,#8316,#291,.T.);
#10323=EDGE_CURVE('',#8315,#8316,#7090,.T.);
#10324=EDGE_CURVE('',#8316,#8297,#1278,.T.);
#10325=EDGE_CURVE('',#8317,#8307,#1279,.T.);
#10326=EDGE_CURVE('',#8317,#8318,#1280,.T.);
#10327=EDGE_CURVE('',#8318,#8308,#1281,.T.);
#10328=EDGE_CURVE('',#8319,#8306,#1282,.T.);
#10329=EDGE_CURVE('',#8319,#8317,#7091,.T.);
#10330=EDGE_CURVE('',#8318,#8320,#7092,.T.);
#10331=EDGE_CURVE('',#8320,#8305,#1283,.T.);
#10332=EDGE_CURVE('',#8320,#8319,#1284,.T.);
#10333=EDGE_CURVE('',#8321,#8322,#292,.T.);
#10334=EDGE_CURVE('',#8321,#8323,#7093,.T.);
#10335=EDGE_CURVE('',#8324,#8323,#293,.T.);
#10336=EDGE_CURVE('',#8324,#8325,#1285,.T.);
#10337=EDGE_CURVE('',#8326,#8325,#294,.T.);
#10338=EDGE_CURVE('',#8327,#8326,#7094,.T.);
#10339=EDGE_CURVE('',#8328,#8327,#295,.T.);
#10340=EDGE_CURVE('',#8328,#8322,#1286,.T.);
#10341=EDGE_CURVE('',#8329,#8330,#1287,.T.);
#10342=EDGE_CURVE('',#8330,#8331,#214,.T.);
#10343=EDGE_CURVE('',#8331,#8332,#1288,.T.);
#10344=EDGE_CURVE('',#8332,#8329,#215,.T.);
#10345=EDGE_CURVE('',#8322,#8333,#1289,.T.);
#10346=EDGE_CURVE('',#8334,#8328,#1290,.T.);
#10347=EDGE_CURVE('',#8333,#8334,#1291,.T.);
#10348=EDGE_CURVE('',#8327,#8335,#1292,.T.);
#10349=EDGE_CURVE('',#8335,#8334,#296,.T.);
#10350=EDGE_CURVE('',#8336,#8326,#1293,.T.);
#10351=EDGE_CURVE('',#8336,#8335,#7095,.T.);
#10352=EDGE_CURVE('',#8337,#8336,#297,.T.);
#10353=EDGE_CURVE('',#8325,#8337,#1294,.T.);
#10354=EDGE_CURVE('',#8338,#8324,#1295,.T.);
#10355=EDGE_CURVE('',#8337,#8338,#1296,.T.);
#10356=EDGE_CURVE('',#8323,#8339,#1297,.T.);
#10357=EDGE_CURVE('',#8339,#8338,#298,.T.);
#10358=EDGE_CURVE('',#8333,#8340,#299,.T.);
#10359=EDGE_CURVE('',#8339,#8340,#7096,.T.);
#10360=EDGE_CURVE('',#8340,#8321,#1298,.T.);
#10361=EDGE_CURVE('',#8341,#8331,#1299,.T.);
#10362=EDGE_CURVE('',#8341,#8342,#1300,.T.);
#10363=EDGE_CURVE('',#8342,#8332,#1301,.T.);
#10364=EDGE_CURVE('',#8343,#8330,#1302,.T.);
#10365=EDGE_CURVE('',#8343,#8341,#7097,.T.);
#10366=EDGE_CURVE('',#8342,#8344,#7098,.T.);
#10367=EDGE_CURVE('',#8344,#8345,#7099,.T.);
#10368=EDGE_CURVE('',#8345,#8346,#7100,.T.);
#10369=EDGE_CURVE('',#8346,#8329,#1303,.T.);
#10370=EDGE_CURVE('',#8346,#8343,#1304,.T.);
#10371=EDGE_CURVE('',#8347,#8348,#1305,.T.);
#10372=EDGE_CURVE('',#8348,#8349,#1306,.T.);
#10373=EDGE_CURVE('',#8349,#8350,#1307,.T.);
#10374=EDGE_CURVE('',#8350,#8351,#1308,.T.);
#10375=EDGE_CURVE('',#8351,#8352,#1309,.T.);
#10376=EDGE_CURVE('',#8352,#8353,#1310,.T.);
#10377=EDGE_CURVE('',#8353,#8354,#1311,.T.);
#10378=EDGE_CURVE('',#8354,#8347,#1312,.T.);
#10379=EDGE_CURVE('',#8355,#8356,#1313,.T.);
#10380=EDGE_CURVE('',#8356,#8357,#1314,.T.);
#10381=EDGE_CURVE('',#8357,#8358,#1315,.T.);
#10382=EDGE_CURVE('',#8358,#8359,#1316,.T.);
#10383=EDGE_CURVE('',#8359,#8360,#1317,.T.);
#10384=EDGE_CURVE('',#8360,#8361,#1318,.T.);
#10385=EDGE_CURVE('',#8361,#8362,#1319,.T.);
#10386=EDGE_CURVE('',#8362,#8355,#1320,.T.);
#10387=EDGE_CURVE('',#8363,#8353,#1321,.T.);
#10388=EDGE_CURVE('',#8352,#8364,#1322,.T.);
#10389=EDGE_CURVE('',#8363,#8364,#1323,.T.);
#10390=EDGE_CURVE('',#8365,#8354,#1324,.T.);
#10391=EDGE_CURVE('',#8365,#8363,#1325,.T.);
#10392=EDGE_CURVE('',#8366,#8367,#1326,.T.);
#10393=EDGE_CURVE('',#8367,#8347,#1327,.T.);
#10394=EDGE_CURVE('',#8366,#8365,#1328,.T.);
#10395=EDGE_CURVE('',#8368,#8349,#1329,.T.);
#10396=EDGE_CURVE('',#8369,#8348,#1330,.T.);
#10397=EDGE_CURVE('',#8370,#8369,#1331,.T.);
#10398=EDGE_CURVE('',#8368,#8370,#1332,.T.);
#10399=EDGE_CURVE('',#8371,#8350,#1333,.T.);
#10400=EDGE_CURVE('',#8371,#8368,#1334,.T.);
#10401=EDGE_CURVE('',#8372,#8351,#1335,.T.);
#10402=EDGE_CURVE('',#8372,#8371,#1336,.T.);
#10403=EDGE_CURVE('',#8364,#8372,#1337,.T.);
#10404=EDGE_CURVE('',#8370,#8373,#1338,.T.);
#10405=EDGE_CURVE('',#8374,#8373,#1339,.T.);
#10406=EDGE_CURVE('',#8366,#8374,#1340,.T.);
#10407=EDGE_CURVE('',#8375,#8376,#1341,.T.);
#10408=EDGE_CURVE('',#8376,#8377,#1342,.T.);
#10409=EDGE_CURVE('',#8377,#8378,#1343,.T.);
#10410=EDGE_CURVE('',#8378,#8379,#1344,.T.);
#10411=EDGE_CURVE('',#8379,#8380,#1345,.T.);
#10412=EDGE_CURVE('',#8380,#8381,#1346,.T.);
#10413=EDGE_CURVE('',#8381,#8382,#1347,.T.);
#10414=EDGE_CURVE('',#8382,#8383,#1348,.T.);
#10415=EDGE_CURVE('',#8383,#8384,#1349,.T.);
#10416=EDGE_CURVE('',#8384,#8385,#1350,.T.);
#10417=EDGE_CURVE('',#8385,#8386,#1351,.T.);
#10418=EDGE_CURVE('',#8386,#8375,#1352,.T.);
#10419=EDGE_CURVE('',#8384,#8356,#1353,.T.);
#10420=EDGE_CURVE('',#8383,#8357,#1354,.T.);
#10421=EDGE_CURVE('',#8358,#8382,#1355,.T.);
#10422=EDGE_CURVE('',#8381,#8359,#1356,.T.);
#10423=EDGE_CURVE('',#8380,#8360,#1357,.T.);
#10424=EDGE_CURVE('',#8379,#8361,#1358,.T.);
#10425=EDGE_CURVE('',#8378,#8362,#1359,.T.);
#10426=EDGE_CURVE('',#8377,#8355,#1360,.T.);
#10427=EDGE_CURVE('',#8387,#8344,#1361,.T.);
#10428=EDGE_CURVE('',#8388,#8387,#1362,.T.);
#10429=EDGE_CURVE('',#8389,#8388,#1363,.T.);
#10430=EDGE_CURVE('',#8389,#8390,#1364,.T.);
#10431=EDGE_CURVE('',#8345,#8390,#1365,.T.);
#10432=EDGE_CURVE('',#8344,#8345,#1366,.T.);
#10433=EDGE_CURVE('',#8391,#8392,#1367,.T.);
#10434=EDGE_CURVE('',#8393,#8391,#1368,.T.);
#10435=EDGE_CURVE('',#8388,#8393,#1369,.T.);
#10436=EDGE_CURVE('',#8376,#8387,#1370,.T.);
#10437=EDGE_CURVE('',#8375,#8392,#1371,.T.);
#10438=EDGE_CURVE('',#8389,#8394,#1372,.T.);
#10439=EDGE_CURVE('',#8395,#8394,#1373,.T.);
#10440=EDGE_CURVE('',#8395,#8396,#1374,.T.);
#10441=EDGE_CURVE('',#8386,#8396,#1375,.T.);
#10442=EDGE_CURVE('',#8390,#8385,#1376,.T.);
#10443=EDGE_CURVE('',#8397,#8393,#1377,.T.);
#10444=EDGE_CURVE('',#8391,#8395,#1378,.T.);
#10445=EDGE_CURVE('',#8394,#8398,#1379,.T.);
#10446=EDGE_CURVE('',#8398,#8374,#1380,.T.);
#10447=EDGE_CURVE('',#8373,#8397,#1381,.T.);
#10448=EDGE_CURVE('',#8388,#8369,#1382,.T.);
#10449=EDGE_CURVE('',#8369,#8397,#1383,.T.);
#10450=EDGE_CURVE('',#8367,#8389,#1384,.T.);
#10451=EDGE_CURVE('',#8367,#8398,#1385,.T.);
#10452=EDGE_CURVE('',#8392,#8396,#1386,.T.);
#13046=ORIENTED_EDGE('',*,*,#10081,.F.);
#13047=ORIENTED_EDGE('',*,*,#10082,.T.);
#13048=ORIENTED_EDGE('',*,*,#10083,.F.);
#13049=ORIENTED_EDGE('',*,*,#10084,.T.);
#13050=ORIENTED_EDGE('',*,*,#10085,.F.);
#13051=ORIENTED_EDGE('',*,*,#10086,.F.);
#13052=ORIENTED_EDGE('',*,*,#10087,.F.);
#13053=ORIENTED_EDGE('',*,*,#10088,.T.);
#13054=ORIENTED_EDGE('',*,*,#10089,.T.);
#13055=ORIENTED_EDGE('',*,*,#10090,.T.);
#13056=ORIENTED_EDGE('',*,*,#10091,.T.);
#13057=ORIENTED_EDGE('',*,*,#10092,.T.);
#13058=ORIENTED_EDGE('',*,*,#10093,.F.);
#13059=ORIENTED_EDGE('',*,*,#10088,.F.);
#13060=ORIENTED_EDGE('',*,*,#10094,.F.);
#13061=ORIENTED_EDGE('',*,*,#10095,.F.);
#13062=ORIENTED_EDGE('',*,*,#10087,.T.);
#13063=ORIENTED_EDGE('',*,*,#10096,.T.);
#13064=ORIENTED_EDGE('',*,*,#10097,.T.);
#13065=ORIENTED_EDGE('',*,*,#10094,.T.);
#13066=ORIENTED_EDGE('',*,*,#10098,.F.);
#13067=ORIENTED_EDGE('',*,*,#10099,.T.);
#13068=ORIENTED_EDGE('',*,*,#10096,.F.);
#13069=ORIENTED_EDGE('',*,*,#10086,.T.);
#13070=ORIENTED_EDGE('',*,*,#10100,.T.);
#13071=ORIENTED_EDGE('',*,*,#10098,.T.);
#13072=ORIENTED_EDGE('',*,*,#10085,.T.);
#13073=ORIENTED_EDGE('',*,*,#10101,.T.);
#13074=ORIENTED_EDGE('',*,*,#10102,.F.);
#13075=ORIENTED_EDGE('',*,*,#10103,.F.);
#13076=ORIENTED_EDGE('',*,*,#10101,.F.);
#13077=ORIENTED_EDGE('',*,*,#10084,.F.);
#13078=ORIENTED_EDGE('',*,*,#10083,.T.);
#13079=ORIENTED_EDGE('',*,*,#10104,.T.);
#13080=ORIENTED_EDGE('',*,*,#10105,.T.);
#13081=ORIENTED_EDGE('',*,*,#10102,.T.);
#13082=ORIENTED_EDGE('',*,*,#10106,.F.);
#13083=ORIENTED_EDGE('',*,*,#10095,.T.);
#13084=ORIENTED_EDGE('',*,*,#10097,.F.);
#13085=ORIENTED_EDGE('',*,*,#10099,.F.);
#13086=ORIENTED_EDGE('',*,*,#10100,.F.);
#13087=ORIENTED_EDGE('',*,*,#10103,.T.);
#13088=ORIENTED_EDGE('',*,*,#10105,.F.);
#13089=ORIENTED_EDGE('',*,*,#10107,.T.);
#13090=ORIENTED_EDGE('',*,*,#10108,.F.);
#13091=ORIENTED_EDGE('',*,*,#10107,.F.);
#13092=ORIENTED_EDGE('',*,*,#10104,.F.);
#13093=ORIENTED_EDGE('',*,*,#10082,.F.);
#13094=ORIENTED_EDGE('',*,*,#10106,.T.);
#13095=ORIENTED_EDGE('',*,*,#10108,.T.);
#13096=ORIENTED_EDGE('',*,*,#10081,.T.);
#13097=ORIENTED_EDGE('',*,*,#10093,.T.);
#13098=ORIENTED_EDGE('',*,*,#10091,.F.);
#13099=ORIENTED_EDGE('',*,*,#10109,.F.);
#13100=ORIENTED_EDGE('',*,*,#10110,.T.);
#13101=ORIENTED_EDGE('',*,*,#10111,.T.);
#13102=ORIENTED_EDGE('',*,*,#10090,.F.);
#13103=ORIENTED_EDGE('',*,*,#10112,.F.);
#13104=ORIENTED_EDGE('',*,*,#10113,.T.);
#13105=ORIENTED_EDGE('',*,*,#10109,.T.);
#13106=ORIENTED_EDGE('',*,*,#10092,.F.);
#13107=ORIENTED_EDGE('',*,*,#10111,.F.);
#13108=ORIENTED_EDGE('',*,*,#10114,.T.);
#13109=ORIENTED_EDGE('',*,*,#10115,.T.);
#13110=ORIENTED_EDGE('',*,*,#10089,.F.);
#13111=ORIENTED_EDGE('',*,*,#10115,.F.);
#13112=ORIENTED_EDGE('',*,*,#10116,.T.);
#13113=ORIENTED_EDGE('',*,*,#10112,.T.);
#13114=ORIENTED_EDGE('',*,*,#10117,.F.);
#13115=ORIENTED_EDGE('',*,*,#10118,.T.);
#13116=ORIENTED_EDGE('',*,*,#10119,.F.);
#13117=ORIENTED_EDGE('',*,*,#10120,.T.);
#13118=ORIENTED_EDGE('',*,*,#10121,.F.);
#13119=ORIENTED_EDGE('',*,*,#10122,.F.);
#13120=ORIENTED_EDGE('',*,*,#10123,.F.);
#13121=ORIENTED_EDGE('',*,*,#10124,.T.);
#13122=ORIENTED_EDGE('',*,*,#10125,.T.);
#13123=ORIENTED_EDGE('',*,*,#10126,.T.);
#13124=ORIENTED_EDGE('',*,*,#10127,.T.);
#13125=ORIENTED_EDGE('',*,*,#10128,.T.);
#13126=ORIENTED_EDGE('',*,*,#10129,.F.);
#13127=ORIENTED_EDGE('',*,*,#10124,.F.);
#13128=ORIENTED_EDGE('',*,*,#10130,.F.);
#13129=ORIENTED_EDGE('',*,*,#10131,.F.);
#13130=ORIENTED_EDGE('',*,*,#10123,.T.);
#13131=ORIENTED_EDGE('',*,*,#10132,.T.);
#13132=ORIENTED_EDGE('',*,*,#10133,.T.);
#13133=ORIENTED_EDGE('',*,*,#10130,.T.);
#13134=ORIENTED_EDGE('',*,*,#10134,.F.);
#13135=ORIENTED_EDGE('',*,*,#10135,.T.);
#13136=ORIENTED_EDGE('',*,*,#10132,.F.);
#13137=ORIENTED_EDGE('',*,*,#10122,.T.);
#13138=ORIENTED_EDGE('',*,*,#10136,.T.);
#13139=ORIENTED_EDGE('',*,*,#10134,.T.);
#13140=ORIENTED_EDGE('',*,*,#10121,.T.);
#13141=ORIENTED_EDGE('',*,*,#10137,.T.);
#13142=ORIENTED_EDGE('',*,*,#10138,.F.);
#13143=ORIENTED_EDGE('',*,*,#10139,.F.);
#13144=ORIENTED_EDGE('',*,*,#10137,.F.);
#13145=ORIENTED_EDGE('',*,*,#10120,.F.);
#13146=ORIENTED_EDGE('',*,*,#10119,.T.);
#13147=ORIENTED_EDGE('',*,*,#10140,.T.);
#13148=ORIENTED_EDGE('',*,*,#10141,.T.);
#13149=ORIENTED_EDGE('',*,*,#10138,.T.);
#13150=ORIENTED_EDGE('',*,*,#10142,.F.);
#13151=ORIENTED_EDGE('',*,*,#10131,.T.);
#13152=ORIENTED_EDGE('',*,*,#10133,.F.);
#13153=ORIENTED_EDGE('',*,*,#10135,.F.);
#13154=ORIENTED_EDGE('',*,*,#10136,.F.);
#13155=ORIENTED_EDGE('',*,*,#10139,.T.);
#13156=ORIENTED_EDGE('',*,*,#10141,.F.);
#13157=ORIENTED_EDGE('',*,*,#10143,.T.);
#13158=ORIENTED_EDGE('',*,*,#10144,.F.);
#13159=ORIENTED_EDGE('',*,*,#10143,.F.);
#13160=ORIENTED_EDGE('',*,*,#10140,.F.);
#13161=ORIENTED_EDGE('',*,*,#10118,.F.);
#13162=ORIENTED_EDGE('',*,*,#10142,.T.);
#13163=ORIENTED_EDGE('',*,*,#10144,.T.);
#13164=ORIENTED_EDGE('',*,*,#10117,.T.);
#13165=ORIENTED_EDGE('',*,*,#10129,.T.);
#13166=ORIENTED_EDGE('',*,*,#10127,.F.);
#13167=ORIENTED_EDGE('',*,*,#10145,.F.);
#13168=ORIENTED_EDGE('',*,*,#10146,.T.);
#13169=ORIENTED_EDGE('',*,*,#10147,.T.);
#13170=ORIENTED_EDGE('',*,*,#10126,.F.);
#13171=ORIENTED_EDGE('',*,*,#10148,.F.);
#13172=ORIENTED_EDGE('',*,*,#10149,.T.);
#13173=ORIENTED_EDGE('',*,*,#10145,.T.);
#13174=ORIENTED_EDGE('',*,*,#10128,.F.);
#13175=ORIENTED_EDGE('',*,*,#10147,.F.);
#13176=ORIENTED_EDGE('',*,*,#10150,.T.);
#13177=ORIENTED_EDGE('',*,*,#10151,.T.);
#13178=ORIENTED_EDGE('',*,*,#10125,.F.);
#13179=ORIENTED_EDGE('',*,*,#10151,.F.);
#13180=ORIENTED_EDGE('',*,*,#10152,.T.);
#13181=ORIENTED_EDGE('',*,*,#10148,.T.);
#13182=ORIENTED_EDGE('',*,*,#10153,.F.);
#13183=ORIENTED_EDGE('',*,*,#10154,.T.);
#13184=ORIENTED_EDGE('',*,*,#10155,.F.);
#13185=ORIENTED_EDGE('',*,*,#10156,.T.);
#13186=ORIENTED_EDGE('',*,*,#10157,.F.);
#13187=ORIENTED_EDGE('',*,*,#10158,.F.);
#13188=ORIENTED_EDGE('',*,*,#10159,.F.);
#13189=ORIENTED_EDGE('',*,*,#10160,.T.);
#13190=ORIENTED_EDGE('',*,*,#10161,.T.);
#13191=ORIENTED_EDGE('',*,*,#10162,.T.);
#13192=ORIENTED_EDGE('',*,*,#10163,.T.);
#13193=ORIENTED_EDGE('',*,*,#10164,.T.);
#13194=ORIENTED_EDGE('',*,*,#10165,.F.);
#13195=ORIENTED_EDGE('',*,*,#10160,.F.);
#13196=ORIENTED_EDGE('',*,*,#10166,.F.);
#13197=ORIENTED_EDGE('',*,*,#10167,.F.);
#13198=ORIENTED_EDGE('',*,*,#10159,.T.);
#13199=ORIENTED_EDGE('',*,*,#10168,.T.);
#13200=ORIENTED_EDGE('',*,*,#10169,.T.);
#13201=ORIENTED_EDGE('',*,*,#10166,.T.);
#13202=ORIENTED_EDGE('',*,*,#10170,.F.);
#13203=ORIENTED_EDGE('',*,*,#10171,.T.);
#13204=ORIENTED_EDGE('',*,*,#10168,.F.);
#13205=ORIENTED_EDGE('',*,*,#10158,.T.);
#13206=ORIENTED_EDGE('',*,*,#10172,.T.);
#13207=ORIENTED_EDGE('',*,*,#10170,.T.);
#13208=ORIENTED_EDGE('',*,*,#10157,.T.);
#13209=ORIENTED_EDGE('',*,*,#10173,.T.);
#13210=ORIENTED_EDGE('',*,*,#10174,.F.);
#13211=ORIENTED_EDGE('',*,*,#10175,.F.);
#13212=ORIENTED_EDGE('',*,*,#10173,.F.);
#13213=ORIENTED_EDGE('',*,*,#10156,.F.);
#13214=ORIENTED_EDGE('',*,*,#10155,.T.);
#13215=ORIENTED_EDGE('',*,*,#10176,.T.);
#13216=ORIENTED_EDGE('',*,*,#10177,.T.);
#13217=ORIENTED_EDGE('',*,*,#10174,.T.);
#13218=ORIENTED_EDGE('',*,*,#10178,.F.);
#13219=ORIENTED_EDGE('',*,*,#10167,.T.);
#13220=ORIENTED_EDGE('',*,*,#10169,.F.);
#13221=ORIENTED_EDGE('',*,*,#10171,.F.);
#13222=ORIENTED_EDGE('',*,*,#10172,.F.);
#13223=ORIENTED_EDGE('',*,*,#10175,.T.);
#13224=ORIENTED_EDGE('',*,*,#10177,.F.);
#13225=ORIENTED_EDGE('',*,*,#10179,.T.);
#13226=ORIENTED_EDGE('',*,*,#10180,.F.);
#13227=ORIENTED_EDGE('',*,*,#10179,.F.);
#13228=ORIENTED_EDGE('',*,*,#10176,.F.);
#13229=ORIENTED_EDGE('',*,*,#10154,.F.);
#13230=ORIENTED_EDGE('',*,*,#10178,.T.);
#13231=ORIENTED_EDGE('',*,*,#10180,.T.);
#13232=ORIENTED_EDGE('',*,*,#10153,.T.);
#13233=ORIENTED_EDGE('',*,*,#10165,.T.);
#13234=ORIENTED_EDGE('',*,*,#10163,.F.);
#13235=ORIENTED_EDGE('',*,*,#10181,.F.);
#13236=ORIENTED_EDGE('',*,*,#10182,.T.);
#13237=ORIENTED_EDGE('',*,*,#10183,.T.);
#13238=ORIENTED_EDGE('',*,*,#10162,.F.);
#13239=ORIENTED_EDGE('',*,*,#10184,.F.);
#13240=ORIENTED_EDGE('',*,*,#10185,.T.);
#13241=ORIENTED_EDGE('',*,*,#10181,.T.);
#13242=ORIENTED_EDGE('',*,*,#10164,.F.);
#13243=ORIENTED_EDGE('',*,*,#10183,.F.);
#13244=ORIENTED_EDGE('',*,*,#10186,.T.);
#13245=ORIENTED_EDGE('',*,*,#10187,.T.);
#13246=ORIENTED_EDGE('',*,*,#10161,.F.);
#13247=ORIENTED_EDGE('',*,*,#10187,.F.);
#13248=ORIENTED_EDGE('',*,*,#10188,.T.);
#13249=ORIENTED_EDGE('',*,*,#10184,.T.);
#13250=ORIENTED_EDGE('',*,*,#10189,.F.);
#13251=ORIENTED_EDGE('',*,*,#10190,.T.);
#13252=ORIENTED_EDGE('',*,*,#10191,.F.);
#13253=ORIENTED_EDGE('',*,*,#10192,.T.);
#13254=ORIENTED_EDGE('',*,*,#10193,.F.);
#13255=ORIENTED_EDGE('',*,*,#10194,.F.);
#13256=ORIENTED_EDGE('',*,*,#10195,.F.);
#13257=ORIENTED_EDGE('',*,*,#10196,.T.);
#13258=ORIENTED_EDGE('',*,*,#10197,.T.);
#13259=ORIENTED_EDGE('',*,*,#10198,.T.);
#13260=ORIENTED_EDGE('',*,*,#10199,.T.);
#13261=ORIENTED_EDGE('',*,*,#10200,.T.);
#13262=ORIENTED_EDGE('',*,*,#10201,.F.);
#13263=ORIENTED_EDGE('',*,*,#10196,.F.);
#13264=ORIENTED_EDGE('',*,*,#10202,.F.);
#13265=ORIENTED_EDGE('',*,*,#10203,.F.);
#13266=ORIENTED_EDGE('',*,*,#10195,.T.);
#13267=ORIENTED_EDGE('',*,*,#10204,.T.);
#13268=ORIENTED_EDGE('',*,*,#10205,.T.);
#13269=ORIENTED_EDGE('',*,*,#10202,.T.);
#13270=ORIENTED_EDGE('',*,*,#10206,.F.);
#13271=ORIENTED_EDGE('',*,*,#10207,.T.);
#13272=ORIENTED_EDGE('',*,*,#10204,.F.);
#13273=ORIENTED_EDGE('',*,*,#10194,.T.);
#13274=ORIENTED_EDGE('',*,*,#10208,.T.);
#13275=ORIENTED_EDGE('',*,*,#10206,.T.);
#13276=ORIENTED_EDGE('',*,*,#10193,.T.);
#13277=ORIENTED_EDGE('',*,*,#10209,.T.);
#13278=ORIENTED_EDGE('',*,*,#10210,.F.);
#13279=ORIENTED_EDGE('',*,*,#10211,.F.);
#13280=ORIENTED_EDGE('',*,*,#10209,.F.);
#13281=ORIENTED_EDGE('',*,*,#10192,.F.);
#13282=ORIENTED_EDGE('',*,*,#10191,.T.);
#13283=ORIENTED_EDGE('',*,*,#10212,.T.);
#13284=ORIENTED_EDGE('',*,*,#10213,.T.);
#13285=ORIENTED_EDGE('',*,*,#10210,.T.);
#13286=ORIENTED_EDGE('',*,*,#10214,.F.);
#13287=ORIENTED_EDGE('',*,*,#10203,.T.);
#13288=ORIENTED_EDGE('',*,*,#10205,.F.);
#13289=ORIENTED_EDGE('',*,*,#10207,.F.);
#13290=ORIENTED_EDGE('',*,*,#10208,.F.);
#13291=ORIENTED_EDGE('',*,*,#10211,.T.);
#13292=ORIENTED_EDGE('',*,*,#10213,.F.);
#13293=ORIENTED_EDGE('',*,*,#10215,.T.);
#13294=ORIENTED_EDGE('',*,*,#10216,.F.);
#13295=ORIENTED_EDGE('',*,*,#10215,.F.);
#13296=ORIENTED_EDGE('',*,*,#10212,.F.);
#13297=ORIENTED_EDGE('',*,*,#10190,.F.);
#13298=ORIENTED_EDGE('',*,*,#10214,.T.);
#13299=ORIENTED_EDGE('',*,*,#10216,.T.);
#13300=ORIENTED_EDGE('',*,*,#10189,.T.);
#13301=ORIENTED_EDGE('',*,*,#10201,.T.);
#13302=ORIENTED_EDGE('',*,*,#10199,.F.);
#13303=ORIENTED_EDGE('',*,*,#10217,.F.);
#13304=ORIENTED_EDGE('',*,*,#10218,.T.);
#13305=ORIENTED_EDGE('',*,*,#10219,.T.);
#13306=ORIENTED_EDGE('',*,*,#10198,.F.);
#13307=ORIENTED_EDGE('',*,*,#10220,.F.);
#13308=ORIENTED_EDGE('',*,*,#10221,.T.);
#13309=ORIENTED_EDGE('',*,*,#10217,.T.);
#13310=ORIENTED_EDGE('',*,*,#10200,.F.);
#13311=ORIENTED_EDGE('',*,*,#10219,.F.);
#13312=ORIENTED_EDGE('',*,*,#10222,.T.);
#13313=ORIENTED_EDGE('',*,*,#10223,.T.);
#13314=ORIENTED_EDGE('',*,*,#10197,.F.);
#13315=ORIENTED_EDGE('',*,*,#10223,.F.);
#13316=ORIENTED_EDGE('',*,*,#10224,.T.);
#13317=ORIENTED_EDGE('',*,*,#10220,.T.);
#13318=ORIENTED_EDGE('',*,*,#10225,.F.);
#13319=ORIENTED_EDGE('',*,*,#10226,.T.);
#13320=ORIENTED_EDGE('',*,*,#10227,.F.);
#13321=ORIENTED_EDGE('',*,*,#10228,.T.);
#13322=ORIENTED_EDGE('',*,*,#10229,.F.);
#13323=ORIENTED_EDGE('',*,*,#10230,.F.);
#13324=ORIENTED_EDGE('',*,*,#10231,.F.);
#13325=ORIENTED_EDGE('',*,*,#10232,.T.);
#13326=ORIENTED_EDGE('',*,*,#10233,.T.);
#13327=ORIENTED_EDGE('',*,*,#10234,.T.);
#13328=ORIENTED_EDGE('',*,*,#10235,.T.);
#13329=ORIENTED_EDGE('',*,*,#10236,.T.);
#13330=ORIENTED_EDGE('',*,*,#10237,.F.);
#13331=ORIENTED_EDGE('',*,*,#10232,.F.);
#13332=ORIENTED_EDGE('',*,*,#10238,.F.);
#13333=ORIENTED_EDGE('',*,*,#10239,.F.);
#13334=ORIENTED_EDGE('',*,*,#10231,.T.);
#13335=ORIENTED_EDGE('',*,*,#10240,.T.);
#13336=ORIENTED_EDGE('',*,*,#10241,.T.);
#13337=ORIENTED_EDGE('',*,*,#10238,.T.);
#13338=ORIENTED_EDGE('',*,*,#10242,.F.);
#13339=ORIENTED_EDGE('',*,*,#10243,.T.);
#13340=ORIENTED_EDGE('',*,*,#10240,.F.);
#13341=ORIENTED_EDGE('',*,*,#10230,.T.);
#13342=ORIENTED_EDGE('',*,*,#10244,.T.);
#13343=ORIENTED_EDGE('',*,*,#10242,.T.);
#13344=ORIENTED_EDGE('',*,*,#10229,.T.);
#13345=ORIENTED_EDGE('',*,*,#10245,.T.);
#13346=ORIENTED_EDGE('',*,*,#10246,.F.);
#13347=ORIENTED_EDGE('',*,*,#10247,.F.);
#13348=ORIENTED_EDGE('',*,*,#10245,.F.);
#13349=ORIENTED_EDGE('',*,*,#10228,.F.);
#13350=ORIENTED_EDGE('',*,*,#10227,.T.);
#13351=ORIENTED_EDGE('',*,*,#10248,.T.);
#13352=ORIENTED_EDGE('',*,*,#10249,.T.);
#13353=ORIENTED_EDGE('',*,*,#10246,.T.);
#13354=ORIENTED_EDGE('',*,*,#10250,.F.);
#13355=ORIENTED_EDGE('',*,*,#10239,.T.);
#13356=ORIENTED_EDGE('',*,*,#10241,.F.);
#13357=ORIENTED_EDGE('',*,*,#10243,.F.);
#13358=ORIENTED_EDGE('',*,*,#10244,.F.);
#13359=ORIENTED_EDGE('',*,*,#10247,.T.);
#13360=ORIENTED_EDGE('',*,*,#10249,.F.);
#13361=ORIENTED_EDGE('',*,*,#10251,.T.);
#13362=ORIENTED_EDGE('',*,*,#10252,.F.);
#13363=ORIENTED_EDGE('',*,*,#10251,.F.);
#13364=ORIENTED_EDGE('',*,*,#10248,.F.);
#13365=ORIENTED_EDGE('',*,*,#10226,.F.);
#13366=ORIENTED_EDGE('',*,*,#10250,.T.);
#13367=ORIENTED_EDGE('',*,*,#10252,.T.);
#13368=ORIENTED_EDGE('',*,*,#10225,.T.);
#13369=ORIENTED_EDGE('',*,*,#10237,.T.);
#13370=ORIENTED_EDGE('',*,*,#10235,.F.);
#13371=ORIENTED_EDGE('',*,*,#10253,.F.);
#13372=ORIENTED_EDGE('',*,*,#10254,.T.);
#13373=ORIENTED_EDGE('',*,*,#10255,.T.);
#13374=ORIENTED_EDGE('',*,*,#10234,.F.);
#13375=ORIENTED_EDGE('',*,*,#10256,.F.);
#13376=ORIENTED_EDGE('',*,*,#10257,.T.);
#13377=ORIENTED_EDGE('',*,*,#10253,.T.);
#13378=ORIENTED_EDGE('',*,*,#10236,.F.);
#13379=ORIENTED_EDGE('',*,*,#10255,.F.);
#13380=ORIENTED_EDGE('',*,*,#10258,.T.);
#13381=ORIENTED_EDGE('',*,*,#10259,.T.);
#13382=ORIENTED_EDGE('',*,*,#10233,.F.);
#13383=ORIENTED_EDGE('',*,*,#10259,.F.);
#13384=ORIENTED_EDGE('',*,*,#10260,.T.);
#13385=ORIENTED_EDGE('',*,*,#10256,.T.);
#13386=ORIENTED_EDGE('',*,*,#10261,.F.);
#13387=ORIENTED_EDGE('',*,*,#10262,.T.);
#13388=ORIENTED_EDGE('',*,*,#10263,.F.);
#13389=ORIENTED_EDGE('',*,*,#10264,.T.);
#13390=ORIENTED_EDGE('',*,*,#10265,.F.);
#13391=ORIENTED_EDGE('',*,*,#10266,.F.);
#13392=ORIENTED_EDGE('',*,*,#10267,.F.);
#13393=ORIENTED_EDGE('',*,*,#10268,.T.);
#13394=ORIENTED_EDGE('',*,*,#10269,.T.);
#13395=ORIENTED_EDGE('',*,*,#10270,.T.);
#13396=ORIENTED_EDGE('',*,*,#10271,.T.);
#13397=ORIENTED_EDGE('',*,*,#10272,.T.);
#13398=ORIENTED_EDGE('',*,*,#10273,.F.);
#13399=ORIENTED_EDGE('',*,*,#10268,.F.);
#13400=ORIENTED_EDGE('',*,*,#10274,.F.);
#13401=ORIENTED_EDGE('',*,*,#10275,.F.);
#13402=ORIENTED_EDGE('',*,*,#10267,.T.);
#13403=ORIENTED_EDGE('',*,*,#10276,.T.);
#13404=ORIENTED_EDGE('',*,*,#10277,.T.);
#13405=ORIENTED_EDGE('',*,*,#10274,.T.);
#13406=ORIENTED_EDGE('',*,*,#10278,.F.);
#13407=ORIENTED_EDGE('',*,*,#10279,.T.);
#13408=ORIENTED_EDGE('',*,*,#10276,.F.);
#13409=ORIENTED_EDGE('',*,*,#10266,.T.);
#13410=ORIENTED_EDGE('',*,*,#10280,.T.);
#13411=ORIENTED_EDGE('',*,*,#10278,.T.);
#13412=ORIENTED_EDGE('',*,*,#10265,.T.);
#13413=ORIENTED_EDGE('',*,*,#10281,.T.);
#13414=ORIENTED_EDGE('',*,*,#10282,.F.);
#13415=ORIENTED_EDGE('',*,*,#10283,.F.);
#13416=ORIENTED_EDGE('',*,*,#10281,.F.);
#13417=ORIENTED_EDGE('',*,*,#10264,.F.);
#13418=ORIENTED_EDGE('',*,*,#10263,.T.);
#13419=ORIENTED_EDGE('',*,*,#10284,.T.);
#13420=ORIENTED_EDGE('',*,*,#10285,.T.);
#13421=ORIENTED_EDGE('',*,*,#10282,.T.);
#13422=ORIENTED_EDGE('',*,*,#10286,.F.);
#13423=ORIENTED_EDGE('',*,*,#10275,.T.);
#13424=ORIENTED_EDGE('',*,*,#10277,.F.);
#13425=ORIENTED_EDGE('',*,*,#10279,.F.);
#13426=ORIENTED_EDGE('',*,*,#10280,.F.);
#13427=ORIENTED_EDGE('',*,*,#10283,.T.);
#13428=ORIENTED_EDGE('',*,*,#10285,.F.);
#13429=ORIENTED_EDGE('',*,*,#10287,.T.);
#13430=ORIENTED_EDGE('',*,*,#10288,.F.);
#13431=ORIENTED_EDGE('',*,*,#10287,.F.);
#13432=ORIENTED_EDGE('',*,*,#10284,.F.);
#13433=ORIENTED_EDGE('',*,*,#10262,.F.);
#13434=ORIENTED_EDGE('',*,*,#10286,.T.);
#13435=ORIENTED_EDGE('',*,*,#10288,.T.);
#13436=ORIENTED_EDGE('',*,*,#10261,.T.);
#13437=ORIENTED_EDGE('',*,*,#10273,.T.);
#13438=ORIENTED_EDGE('',*,*,#10271,.F.);
#13439=ORIENTED_EDGE('',*,*,#10289,.F.);
#13440=ORIENTED_EDGE('',*,*,#10290,.T.);
#13441=ORIENTED_EDGE('',*,*,#10291,.T.);
#13442=ORIENTED_EDGE('',*,*,#10270,.F.);
#13443=ORIENTED_EDGE('',*,*,#10292,.F.);
#13444=ORIENTED_EDGE('',*,*,#10293,.T.);
#13445=ORIENTED_EDGE('',*,*,#10289,.T.);
#13446=ORIENTED_EDGE('',*,*,#10272,.F.);
#13447=ORIENTED_EDGE('',*,*,#10291,.F.);
#13448=ORIENTED_EDGE('',*,*,#10294,.T.);
#13449=ORIENTED_EDGE('',*,*,#10295,.T.);
#13450=ORIENTED_EDGE('',*,*,#10269,.F.);
#13451=ORIENTED_EDGE('',*,*,#10295,.F.);
#13452=ORIENTED_EDGE('',*,*,#10296,.T.);
#13453=ORIENTED_EDGE('',*,*,#10292,.T.);
#13454=ORIENTED_EDGE('',*,*,#10297,.F.);
#13455=ORIENTED_EDGE('',*,*,#10298,.T.);
#13456=ORIENTED_EDGE('',*,*,#10299,.F.);
#13457=ORIENTED_EDGE('',*,*,#10300,.T.);
#13458=ORIENTED_EDGE('',*,*,#10301,.F.);
#13459=ORIENTED_EDGE('',*,*,#10302,.F.);
#13460=ORIENTED_EDGE('',*,*,#10303,.F.);
#13461=ORIENTED_EDGE('',*,*,#10304,.T.);
#13462=ORIENTED_EDGE('',*,*,#10305,.T.);
#13463=ORIENTED_EDGE('',*,*,#10306,.T.);
#13464=ORIENTED_EDGE('',*,*,#10307,.T.);
#13465=ORIENTED_EDGE('',*,*,#10308,.T.);
#13466=ORIENTED_EDGE('',*,*,#10309,.F.);
#13467=ORIENTED_EDGE('',*,*,#10304,.F.);
#13468=ORIENTED_EDGE('',*,*,#10310,.F.);
#13469=ORIENTED_EDGE('',*,*,#10311,.F.);
#13470=ORIENTED_EDGE('',*,*,#10303,.T.);
#13471=ORIENTED_EDGE('',*,*,#10312,.T.);
#13472=ORIENTED_EDGE('',*,*,#10313,.T.);
#13473=ORIENTED_EDGE('',*,*,#10310,.T.);
#13474=ORIENTED_EDGE('',*,*,#10314,.F.);
#13475=ORIENTED_EDGE('',*,*,#10315,.T.);
#13476=ORIENTED_EDGE('',*,*,#10312,.F.);
#13477=ORIENTED_EDGE('',*,*,#10302,.T.);
#13478=ORIENTED_EDGE('',*,*,#10316,.T.);
#13479=ORIENTED_EDGE('',*,*,#10314,.T.);
#13480=ORIENTED_EDGE('',*,*,#10301,.T.);
#13481=ORIENTED_EDGE('',*,*,#10317,.T.);
#13482=ORIENTED_EDGE('',*,*,#10318,.F.);
#13483=ORIENTED_EDGE('',*,*,#10319,.F.);
#13484=ORIENTED_EDGE('',*,*,#10317,.F.);
#13485=ORIENTED_EDGE('',*,*,#10300,.F.);
#13486=ORIENTED_EDGE('',*,*,#10299,.T.);
#13487=ORIENTED_EDGE('',*,*,#10320,.T.);
#13488=ORIENTED_EDGE('',*,*,#10321,.T.);
#13489=ORIENTED_EDGE('',*,*,#10318,.T.);
#13490=ORIENTED_EDGE('',*,*,#10322,.F.);
#13491=ORIENTED_EDGE('',*,*,#10311,.T.);
#13492=ORIENTED_EDGE('',*,*,#10313,.F.);
#13493=ORIENTED_EDGE('',*,*,#10315,.F.);
#13494=ORIENTED_EDGE('',*,*,#10316,.F.);
#13495=ORIENTED_EDGE('',*,*,#10319,.T.);
#13496=ORIENTED_EDGE('',*,*,#10321,.F.);
#13497=ORIENTED_EDGE('',*,*,#10323,.T.);
#13498=ORIENTED_EDGE('',*,*,#10324,.F.);
#13499=ORIENTED_EDGE('',*,*,#10323,.F.);
#13500=ORIENTED_EDGE('',*,*,#10320,.F.);
#13501=ORIENTED_EDGE('',*,*,#10298,.F.);
#13502=ORIENTED_EDGE('',*,*,#10322,.T.);
#13503=ORIENTED_EDGE('',*,*,#10324,.T.);
#13504=ORIENTED_EDGE('',*,*,#10297,.T.);
#13505=ORIENTED_EDGE('',*,*,#10309,.T.);
#13506=ORIENTED_EDGE('',*,*,#10307,.F.);
#13507=ORIENTED_EDGE('',*,*,#10325,.F.);
#13508=ORIENTED_EDGE('',*,*,#10326,.T.);
#13509=ORIENTED_EDGE('',*,*,#10327,.T.);
#13510=ORIENTED_EDGE('',*,*,#10306,.F.);
#13511=ORIENTED_EDGE('',*,*,#10328,.F.);
#13512=ORIENTED_EDGE('',*,*,#10329,.T.);
#13513=ORIENTED_EDGE('',*,*,#10325,.T.);
#13514=ORIENTED_EDGE('',*,*,#10308,.F.);
#13515=ORIENTED_EDGE('',*,*,#10327,.F.);
#13516=ORIENTED_EDGE('',*,*,#10330,.T.);
#13517=ORIENTED_EDGE('',*,*,#10331,.T.);
#13518=ORIENTED_EDGE('',*,*,#10305,.F.);
#13519=ORIENTED_EDGE('',*,*,#10331,.F.);
#13520=ORIENTED_EDGE('',*,*,#10332,.T.);
#13521=ORIENTED_EDGE('',*,*,#10328,.T.);
#13522=ORIENTED_EDGE('',*,*,#10333,.F.);
#13523=ORIENTED_EDGE('',*,*,#10334,.T.);
#13524=ORIENTED_EDGE('',*,*,#10335,.F.);
#13525=ORIENTED_EDGE('',*,*,#10336,.T.);
#13526=ORIENTED_EDGE('',*,*,#10337,.F.);
#13527=ORIENTED_EDGE('',*,*,#10338,.F.);
#13528=ORIENTED_EDGE('',*,*,#10339,.F.);
#13529=ORIENTED_EDGE('',*,*,#10340,.T.);
#13530=ORIENTED_EDGE('',*,*,#10341,.T.);
#13531=ORIENTED_EDGE('',*,*,#10342,.T.);
#13532=ORIENTED_EDGE('',*,*,#10343,.T.);
#13533=ORIENTED_EDGE('',*,*,#10344,.T.);
#13534=ORIENTED_EDGE('',*,*,#10345,.F.);
#13535=ORIENTED_EDGE('',*,*,#10340,.F.);
#13536=ORIENTED_EDGE('',*,*,#10346,.F.);
#13537=ORIENTED_EDGE('',*,*,#10347,.F.);
#13538=ORIENTED_EDGE('',*,*,#10339,.T.);
#13539=ORIENTED_EDGE('',*,*,#10348,.T.);
#13540=ORIENTED_EDGE('',*,*,#10349,.T.);
#13541=ORIENTED_EDGE('',*,*,#10346,.T.);
#13542=ORIENTED_EDGE('',*,*,#10350,.F.);
#13543=ORIENTED_EDGE('',*,*,#10351,.T.);
#13544=ORIENTED_EDGE('',*,*,#10348,.F.);
#13545=ORIENTED_EDGE('',*,*,#10338,.T.);
#13546=ORIENTED_EDGE('',*,*,#10352,.T.);
#13547=ORIENTED_EDGE('',*,*,#10350,.T.);
#13548=ORIENTED_EDGE('',*,*,#10337,.T.);
#13549=ORIENTED_EDGE('',*,*,#10353,.T.);
#13550=ORIENTED_EDGE('',*,*,#10354,.F.);
#13551=ORIENTED_EDGE('',*,*,#10355,.F.);
#13552=ORIENTED_EDGE('',*,*,#10353,.F.);
#13553=ORIENTED_EDGE('',*,*,#10336,.F.);
#13554=ORIENTED_EDGE('',*,*,#10335,.T.);
#13555=ORIENTED_EDGE('',*,*,#10356,.T.);
#13556=ORIENTED_EDGE('',*,*,#10357,.T.);
#13557=ORIENTED_EDGE('',*,*,#10354,.T.);
#13558=ORIENTED_EDGE('',*,*,#10358,.F.);
#13559=ORIENTED_EDGE('',*,*,#10347,.T.);
#13560=ORIENTED_EDGE('',*,*,#10349,.F.);
#13561=ORIENTED_EDGE('',*,*,#10351,.F.);
#13562=ORIENTED_EDGE('',*,*,#10352,.F.);
#13563=ORIENTED_EDGE('',*,*,#10355,.T.);
#13564=ORIENTED_EDGE('',*,*,#10357,.F.);
#13565=ORIENTED_EDGE('',*,*,#10359,.T.);
#13566=ORIENTED_EDGE('',*,*,#10360,.F.);
#13567=ORIENTED_EDGE('',*,*,#10359,.F.);
#13568=ORIENTED_EDGE('',*,*,#10356,.F.);
#13569=ORIENTED_EDGE('',*,*,#10334,.F.);
#13570=ORIENTED_EDGE('',*,*,#10358,.T.);
#13571=ORIENTED_EDGE('',*,*,#10360,.T.);
#13572=ORIENTED_EDGE('',*,*,#10333,.T.);
#13573=ORIENTED_EDGE('',*,*,#10345,.T.);
#13574=ORIENTED_EDGE('',*,*,#10343,.F.);
#13575=ORIENTED_EDGE('',*,*,#10361,.F.);
#13576=ORIENTED_EDGE('',*,*,#10362,.T.);
#13577=ORIENTED_EDGE('',*,*,#10363,.T.);
#13578=ORIENTED_EDGE('',*,*,#10342,.F.);
#13579=ORIENTED_EDGE('',*,*,#10364,.F.);
#13580=ORIENTED_EDGE('',*,*,#10365,.T.);
#13581=ORIENTED_EDGE('',*,*,#10361,.T.);
#13582=ORIENTED_EDGE('',*,*,#10344,.F.);
#13583=ORIENTED_EDGE('',*,*,#10363,.F.);
#13584=ORIENTED_EDGE('',*,*,#10366,.T.);
#13585=ORIENTED_EDGE('',*,*,#10367,.T.);
#13586=ORIENTED_EDGE('',*,*,#10368,.T.);
#13587=ORIENTED_EDGE('',*,*,#10369,.T.);
#13588=ORIENTED_EDGE('',*,*,#10341,.F.);
#13589=ORIENTED_EDGE('',*,*,#10369,.F.);
#13590=ORIENTED_EDGE('',*,*,#10370,.T.);
#13591=ORIENTED_EDGE('',*,*,#10364,.T.);
#13592=ORIENTED_EDGE('',*,*,#10371,.T.);
#13593=ORIENTED_EDGE('',*,*,#10372,.T.);
#13594=ORIENTED_EDGE('',*,*,#10373,.T.);
#13595=ORIENTED_EDGE('',*,*,#10374,.T.);
#13596=ORIENTED_EDGE('',*,*,#10375,.T.);
#13597=ORIENTED_EDGE('',*,*,#10376,.T.);
#13598=ORIENTED_EDGE('',*,*,#10377,.T.);
#13599=ORIENTED_EDGE('',*,*,#10378,.T.);
#13600=ORIENTED_EDGE('',*,*,#10379,.T.);
#13601=ORIENTED_EDGE('',*,*,#10380,.T.);
#13602=ORIENTED_EDGE('',*,*,#10381,.T.);
#13603=ORIENTED_EDGE('',*,*,#10382,.T.);
#13604=ORIENTED_EDGE('',*,*,#10383,.T.);
#13605=ORIENTED_EDGE('',*,*,#10384,.T.);
#13606=ORIENTED_EDGE('',*,*,#10385,.T.);
#13607=ORIENTED_EDGE('',*,*,#10386,.T.);
#13608=ORIENTED_EDGE('',*,*,#10387,.T.);
#13609=ORIENTED_EDGE('',*,*,#10376,.F.);
#13610=ORIENTED_EDGE('',*,*,#10388,.T.);
#13611=ORIENTED_EDGE('',*,*,#10389,.F.);
#13612=ORIENTED_EDGE('',*,*,#10390,.T.);
#13613=ORIENTED_EDGE('',*,*,#10377,.F.);
#13614=ORIENTED_EDGE('',*,*,#10387,.F.);
#13615=ORIENTED_EDGE('',*,*,#10391,.F.);
#13616=ORIENTED_EDGE('',*,*,#10392,.T.);
#13617=ORIENTED_EDGE('',*,*,#10393,.T.);
#13618=ORIENTED_EDGE('',*,*,#10378,.F.);
#13619=ORIENTED_EDGE('',*,*,#10390,.F.);
#13620=ORIENTED_EDGE('',*,*,#10394,.F.);
#13621=ORIENTED_EDGE('',*,*,#10395,.T.);
#13622=ORIENTED_EDGE('',*,*,#10372,.F.);
#13623=ORIENTED_EDGE('',*,*,#10396,.F.);
#13624=ORIENTED_EDGE('',*,*,#10397,.F.);
#13625=ORIENTED_EDGE('',*,*,#10398,.F.);
#13626=ORIENTED_EDGE('',*,*,#10399,.T.);
#13627=ORIENTED_EDGE('',*,*,#10373,.F.);
#13628=ORIENTED_EDGE('',*,*,#10395,.F.);
#13629=ORIENTED_EDGE('',*,*,#10400,.F.);
#13630=ORIENTED_EDGE('',*,*,#10401,.T.);
#13631=ORIENTED_EDGE('',*,*,#10374,.F.);
#13632=ORIENTED_EDGE('',*,*,#10399,.F.);
#13633=ORIENTED_EDGE('',*,*,#10402,.F.);
#13634=ORIENTED_EDGE('',*,*,#10388,.F.);
#13635=ORIENTED_EDGE('',*,*,#10375,.F.);
#13636=ORIENTED_EDGE('',*,*,#10401,.F.);
#13637=ORIENTED_EDGE('',*,*,#10403,.F.);
#13638=ORIENTED_EDGE('',*,*,#10389,.T.);
#13639=ORIENTED_EDGE('',*,*,#10403,.T.);
#13640=ORIENTED_EDGE('',*,*,#10402,.T.);
#13641=ORIENTED_EDGE('',*,*,#10400,.T.);
#13642=ORIENTED_EDGE('',*,*,#10398,.T.);
#13643=ORIENTED_EDGE('',*,*,#10404,.T.);
#13644=ORIENTED_EDGE('',*,*,#10405,.F.);
#13645=ORIENTED_EDGE('',*,*,#10406,.F.);
#13646=ORIENTED_EDGE('',*,*,#10394,.T.);
#13647=ORIENTED_EDGE('',*,*,#10391,.T.);
#13648=ORIENTED_EDGE('',*,*,#10407,.T.);
#13649=ORIENTED_EDGE('',*,*,#10408,.T.);
#13650=ORIENTED_EDGE('',*,*,#10409,.T.);
#13651=ORIENTED_EDGE('',*,*,#10410,.T.);
#13652=ORIENTED_EDGE('',*,*,#10411,.T.);
#13653=ORIENTED_EDGE('',*,*,#10412,.T.);
#13654=ORIENTED_EDGE('',*,*,#10413,.T.);
#13655=ORIENTED_EDGE('',*,*,#10414,.T.);
#13656=ORIENTED_EDGE('',*,*,#10415,.T.);
#13657=ORIENTED_EDGE('',*,*,#10416,.T.);
#13658=ORIENTED_EDGE('',*,*,#10417,.T.);
#13659=ORIENTED_EDGE('',*,*,#10418,.T.);
#13660=ORIENTED_EDGE('',*,*,#10419,.F.);
#13661=ORIENTED_EDGE('',*,*,#10415,.F.);
#13662=ORIENTED_EDGE('',*,*,#10420,.T.);
#13663=ORIENTED_EDGE('',*,*,#10380,.F.);
#13664=ORIENTED_EDGE('',*,*,#10332,.F.);
#13665=ORIENTED_EDGE('',*,*,#10330,.F.);
#13666=ORIENTED_EDGE('',*,*,#10326,.F.);
#13667=ORIENTED_EDGE('',*,*,#10329,.F.);
#13668=ORIENTED_EDGE('',*,*,#10420,.F.);
#13669=ORIENTED_EDGE('',*,*,#10414,.F.);
#13670=ORIENTED_EDGE('',*,*,#10421,.F.);
#13671=ORIENTED_EDGE('',*,*,#10381,.F.);
#13672=ORIENTED_EDGE('',*,*,#10296,.F.);
#13673=ORIENTED_EDGE('',*,*,#10294,.F.);
#13674=ORIENTED_EDGE('',*,*,#10290,.F.);
#13675=ORIENTED_EDGE('',*,*,#10293,.F.);
#13676=ORIENTED_EDGE('',*,*,#10422,.T.);
#13677=ORIENTED_EDGE('',*,*,#10382,.F.);
#13678=ORIENTED_EDGE('',*,*,#10421,.T.);
#13679=ORIENTED_EDGE('',*,*,#10413,.F.);
#13680=ORIENTED_EDGE('',*,*,#10260,.F.);
#13681=ORIENTED_EDGE('',*,*,#10258,.F.);
#13682=ORIENTED_EDGE('',*,*,#10254,.F.);
#13683=ORIENTED_EDGE('',*,*,#10257,.F.);
#13684=ORIENTED_EDGE('',*,*,#10423,.T.);
#13685=ORIENTED_EDGE('',*,*,#10383,.F.);
#13686=ORIENTED_EDGE('',*,*,#10422,.F.);
#13687=ORIENTED_EDGE('',*,*,#10412,.F.);
#13688=ORIENTED_EDGE('',*,*,#10224,.F.);
#13689=ORIENTED_EDGE('',*,*,#10222,.F.);
#13690=ORIENTED_EDGE('',*,*,#10218,.F.);
#13691=ORIENTED_EDGE('',*,*,#10221,.F.);
#13692=ORIENTED_EDGE('',*,*,#10424,.T.);
#13693=ORIENTED_EDGE('',*,*,#10384,.F.);
#13694=ORIENTED_EDGE('',*,*,#10423,.F.);
#13695=ORIENTED_EDGE('',*,*,#10411,.F.);
#13696=ORIENTED_EDGE('',*,*,#10188,.F.);
#13697=ORIENTED_EDGE('',*,*,#10186,.F.);
#13698=ORIENTED_EDGE('',*,*,#10182,.F.);
#13699=ORIENTED_EDGE('',*,*,#10185,.F.);
#13700=ORIENTED_EDGE('',*,*,#10424,.F.);
#13701=ORIENTED_EDGE('',*,*,#10410,.F.);
#13702=ORIENTED_EDGE('',*,*,#10425,.T.);
#13703=ORIENTED_EDGE('',*,*,#10385,.F.);
#13704=ORIENTED_EDGE('',*,*,#10152,.F.);
#13705=ORIENTED_EDGE('',*,*,#10150,.F.);
#13706=ORIENTED_EDGE('',*,*,#10146,.F.);
#13707=ORIENTED_EDGE('',*,*,#10149,.F.);
#13708=ORIENTED_EDGE('',*,*,#10425,.F.);
#13709=ORIENTED_EDGE('',*,*,#10409,.F.);
#13710=ORIENTED_EDGE('',*,*,#10426,.T.);
#13711=ORIENTED_EDGE('',*,*,#10386,.F.);
#13712=ORIENTED_EDGE('',*,*,#10116,.F.);
#13713=ORIENTED_EDGE('',*,*,#10114,.F.);
#13714=ORIENTED_EDGE('',*,*,#10110,.F.);
#13715=ORIENTED_EDGE('',*,*,#10113,.F.);
#13716=ORIENTED_EDGE('',*,*,#10427,.F.);
#13717=ORIENTED_EDGE('',*,*,#10428,.F.);
#13718=ORIENTED_EDGE('',*,*,#10429,.F.);
#13719=ORIENTED_EDGE('',*,*,#10430,.T.);
#13720=ORIENTED_EDGE('',*,*,#10431,.F.);
#13721=ORIENTED_EDGE('',*,*,#10432,.F.);
#13722=ORIENTED_EDGE('',*,*,#10433,.F.);
#13723=ORIENTED_EDGE('',*,*,#10434,.F.);
#13724=ORIENTED_EDGE('',*,*,#10435,.F.);
#13725=ORIENTED_EDGE('',*,*,#10428,.T.);
#13726=ORIENTED_EDGE('',*,*,#10436,.F.);
#13727=ORIENTED_EDGE('',*,*,#10407,.F.);
#13728=ORIENTED_EDGE('',*,*,#10437,.T.);
#13729=ORIENTED_EDGE('',*,*,#10438,.T.);
#13730=ORIENTED_EDGE('',*,*,#10439,.F.);
#13731=ORIENTED_EDGE('',*,*,#10440,.T.);
#13732=ORIENTED_EDGE('',*,*,#10441,.F.);
#13733=ORIENTED_EDGE('',*,*,#10417,.F.);
#13734=ORIENTED_EDGE('',*,*,#10442,.F.);
#13735=ORIENTED_EDGE('',*,*,#10430,.F.);
#13736=ORIENTED_EDGE('',*,*,#10367,.F.);
#13737=ORIENTED_EDGE('',*,*,#10432,.T.);
#13738=ORIENTED_EDGE('',*,*,#10443,.T.);
#13739=ORIENTED_EDGE('',*,*,#10434,.T.);
#13740=ORIENTED_EDGE('',*,*,#10444,.T.);
#13741=ORIENTED_EDGE('',*,*,#10439,.T.);
#13742=ORIENTED_EDGE('',*,*,#10445,.T.);
#13743=ORIENTED_EDGE('',*,*,#10446,.T.);
#13744=ORIENTED_EDGE('',*,*,#10405,.T.);
#13745=ORIENTED_EDGE('',*,*,#10447,.T.);
#13746=ORIENTED_EDGE('',*,*,#10448,.F.);
#13747=ORIENTED_EDGE('',*,*,#10435,.T.);
#13748=ORIENTED_EDGE('',*,*,#10443,.F.);
#13749=ORIENTED_EDGE('',*,*,#10449,.F.);
#13750=ORIENTED_EDGE('',*,*,#10450,.F.);
#13751=ORIENTED_EDGE('',*,*,#10451,.T.);
#13752=ORIENTED_EDGE('',*,*,#10445,.F.);
#13753=ORIENTED_EDGE('',*,*,#10438,.F.);
#13754=ORIENTED_EDGE('',*,*,#10392,.F.);
#13755=ORIENTED_EDGE('',*,*,#10406,.T.);
#13756=ORIENTED_EDGE('',*,*,#10446,.F.);
#13757=ORIENTED_EDGE('',*,*,#10451,.F.);
#13758=ORIENTED_EDGE('',*,*,#10397,.T.);
#13759=ORIENTED_EDGE('',*,*,#10449,.T.);
#13760=ORIENTED_EDGE('',*,*,#10447,.F.);
#13761=ORIENTED_EDGE('',*,*,#10404,.F.);
#13762=ORIENTED_EDGE('',*,*,#10426,.F.);
#13763=ORIENTED_EDGE('',*,*,#10408,.F.);
#13764=ORIENTED_EDGE('',*,*,#10436,.T.);
#13765=ORIENTED_EDGE('',*,*,#10427,.T.);
#13766=ORIENTED_EDGE('',*,*,#10366,.F.);
#13767=ORIENTED_EDGE('',*,*,#10362,.F.);
#13768=ORIENTED_EDGE('',*,*,#10365,.F.);
#13769=ORIENTED_EDGE('',*,*,#10370,.F.);
#13770=ORIENTED_EDGE('',*,*,#10368,.F.);
#13771=ORIENTED_EDGE('',*,*,#10431,.T.);
#13772=ORIENTED_EDGE('',*,*,#10442,.T.);
#13773=ORIENTED_EDGE('',*,*,#10416,.F.);
#13774=ORIENTED_EDGE('',*,*,#10419,.T.);
#13775=ORIENTED_EDGE('',*,*,#10379,.F.);
#13776=ORIENTED_EDGE('',*,*,#10448,.T.);
#13777=ORIENTED_EDGE('',*,*,#10396,.T.);
#13778=ORIENTED_EDGE('',*,*,#10371,.F.);
#13779=ORIENTED_EDGE('',*,*,#10393,.F.);
#13780=ORIENTED_EDGE('',*,*,#10450,.T.);
#13781=ORIENTED_EDGE('',*,*,#10429,.T.);
#13782=ORIENTED_EDGE('',*,*,#10452,.T.);
#13783=ORIENTED_EDGE('',*,*,#10440,.F.);
#13784=ORIENTED_EDGE('',*,*,#10444,.F.);
#13785=ORIENTED_EDGE('',*,*,#10433,.T.);
#13786=ORIENTED_EDGE('',*,*,#10452,.F.);
#13787=ORIENTED_EDGE('',*,*,#10437,.F.);
#13788=ORIENTED_EDGE('',*,*,#10418,.F.);
#13789=ORIENTED_EDGE('',*,*,#10441,.T.);
#18555=ADVANCED_FACE('',(#4839,#484),#4307,.T.);
#18556=ADVANCED_FACE('',(#4840),#608,.F.);
#18557=ADVANCED_FACE('',(#4841),#609,.T.);
#18558=ADVANCED_FACE('',(#4842),#610,.T.);
#18559=ADVANCED_FACE('',(#4843),#611,.T.);
#18560=ADVANCED_FACE('',(#4844),#612,.F.);
#18561=ADVANCED_FACE('',(#4845),#613,.T.);
#18562=ADVANCED_FACE('',(#4846),#4308,.F.);
#18563=ADVANCED_FACE('',(#4847),#614,.T.);
#18564=ADVANCED_FACE('',(#4848),#615,.T.);
#18565=ADVANCED_FACE('',(#4849),#616,.T.);
#18566=ADVANCED_FACE('',(#4850),#4309,.T.);
#18567=ADVANCED_FACE('',(#4851),#4310,.T.);
#18568=ADVANCED_FACE('',(#4852),#617,.T.);
#18569=ADVANCED_FACE('',(#4853,#485),#4311,.T.);
#18570=ADVANCED_FACE('',(#4854),#618,.F.);
#18571=ADVANCED_FACE('',(#4855),#619,.T.);
#18572=ADVANCED_FACE('',(#4856),#620,.T.);
#18573=ADVANCED_FACE('',(#4857),#621,.T.);
#18574=ADVANCED_FACE('',(#4858),#622,.F.);
#18575=ADVANCED_FACE('',(#4859),#623,.T.);
#18576=ADVANCED_FACE('',(#4860),#4312,.F.);
#18577=ADVANCED_FACE('',(#4861),#624,.T.);
#18578=ADVANCED_FACE('',(#4862),#625,.T.);
#18579=ADVANCED_FACE('',(#4863),#626,.T.);
#18580=ADVANCED_FACE('',(#4864),#4313,.T.);
#18581=ADVANCED_FACE('',(#4865),#4314,.T.);
#18582=ADVANCED_FACE('',(#4866),#627,.T.);
#18583=ADVANCED_FACE('',(#4867,#486),#4315,.T.);
#18584=ADVANCED_FACE('',(#4868),#628,.F.);
#18585=ADVANCED_FACE('',(#4869),#629,.T.);
#18586=ADVANCED_FACE('',(#4870),#630,.T.);
#18587=ADVANCED_FACE('',(#4871),#631,.T.);
#18588=ADVANCED_FACE('',(#4872),#632,.F.);
#18589=ADVANCED_FACE('',(#4873),#633,.T.);
#18590=ADVANCED_FACE('',(#4874),#4316,.F.);
#18591=ADVANCED_FACE('',(#4875),#634,.T.);
#18592=ADVANCED_FACE('',(#4876),#635,.T.);
#18593=ADVANCED_FACE('',(#4877),#636,.T.);
#18594=ADVANCED_FACE('',(#4878),#4317,.T.);
#18595=ADVANCED_FACE('',(#4879),#4318,.T.);
#18596=ADVANCED_FACE('',(#4880),#637,.T.);
#18597=ADVANCED_FACE('',(#4881,#487),#4319,.T.);
#18598=ADVANCED_FACE('',(#4882),#638,.F.);
#18599=ADVANCED_FACE('',(#4883),#639,.T.);
#18600=ADVANCED_FACE('',(#4884),#640,.T.);
#18601=ADVANCED_FACE('',(#4885),#641,.T.);
#18602=ADVANCED_FACE('',(#4886),#642,.F.);
#18603=ADVANCED_FACE('',(#4887),#643,.T.);
#18604=ADVANCED_FACE('',(#4888),#4320,.F.);
#18605=ADVANCED_FACE('',(#4889),#644,.T.);
#18606=ADVANCED_FACE('',(#4890),#645,.T.);
#18607=ADVANCED_FACE('',(#4891),#646,.T.);
#18608=ADVANCED_FACE('',(#4892),#4321,.T.);
#18609=ADVANCED_FACE('',(#4893),#4322,.T.);
#18610=ADVANCED_FACE('',(#4894),#647,.T.);
#18611=ADVANCED_FACE('',(#4895,#488),#4323,.T.);
#18612=ADVANCED_FACE('',(#4896),#648,.F.);
#18613=ADVANCED_FACE('',(#4897),#649,.T.);
#18614=ADVANCED_FACE('',(#4898),#650,.T.);
#18615=ADVANCED_FACE('',(#4899),#651,.T.);
#18616=ADVANCED_FACE('',(#4900),#652,.F.);
#18617=ADVANCED_FACE('',(#4901),#653,.T.);
#18618=ADVANCED_FACE('',(#4902),#4324,.F.);
#18619=ADVANCED_FACE('',(#4903),#654,.T.);
#18620=ADVANCED_FACE('',(#4904),#655,.T.);
#18621=ADVANCED_FACE('',(#4905),#656,.T.);
#18622=ADVANCED_FACE('',(#4906),#4325,.T.);
#18623=ADVANCED_FACE('',(#4907),#4326,.T.);
#18624=ADVANCED_FACE('',(#4908),#657,.T.);
#18625=ADVANCED_FACE('',(#4909,#489),#4327,.T.);
#18626=ADVANCED_FACE('',(#4910),#658,.F.);
#18627=ADVANCED_FACE('',(#4911),#659,.T.);
#18628=ADVANCED_FACE('',(#4912),#660,.T.);
#18629=ADVANCED_FACE('',(#4913),#661,.T.);
#18630=ADVANCED_FACE('',(#4914),#662,.F.);
#18631=ADVANCED_FACE('',(#4915),#663,.T.);
#18632=ADVANCED_FACE('',(#4916),#4328,.F.);
#18633=ADVANCED_FACE('',(#4917),#664,.T.);
#18634=ADVANCED_FACE('',(#4918),#665,.T.);
#18635=ADVANCED_FACE('',(#4919),#666,.T.);
#18636=ADVANCED_FACE('',(#4920),#4329,.T.);
#18637=ADVANCED_FACE('',(#4921),#4330,.T.);
#18638=ADVANCED_FACE('',(#4922),#667,.T.);
#18639=ADVANCED_FACE('',(#4923,#490),#4331,.T.);
#18640=ADVANCED_FACE('',(#4924),#668,.F.);
#18641=ADVANCED_FACE('',(#4925),#669,.T.);
#18642=ADVANCED_FACE('',(#4926),#670,.T.);
#18643=ADVANCED_FACE('',(#4927),#671,.T.);
#18644=ADVANCED_FACE('',(#4928),#672,.F.);
#18645=ADVANCED_FACE('',(#4929),#673,.T.);
#18646=ADVANCED_FACE('',(#4930),#4332,.F.);
#18647=ADVANCED_FACE('',(#4931),#674,.T.);
#18648=ADVANCED_FACE('',(#4932),#675,.T.);
#18649=ADVANCED_FACE('',(#4933),#676,.T.);
#18650=ADVANCED_FACE('',(#4934),#4333,.T.);
#18651=ADVANCED_FACE('',(#4935),#4334,.T.);
#18652=ADVANCED_FACE('',(#4936),#677,.T.);
#18653=ADVANCED_FACE('',(#4937,#491),#4335,.T.);
#18654=ADVANCED_FACE('',(#4938),#678,.F.);
#18655=ADVANCED_FACE('',(#4939),#679,.T.);
#18656=ADVANCED_FACE('',(#4940),#680,.T.);
#18657=ADVANCED_FACE('',(#4941),#681,.T.);
#18658=ADVANCED_FACE('',(#4942),#682,.F.);
#18659=ADVANCED_FACE('',(#4943),#683,.T.);
#18660=ADVANCED_FACE('',(#4944),#4336,.F.);
#18661=ADVANCED_FACE('',(#4945),#684,.T.);
#18662=ADVANCED_FACE('',(#4946),#685,.T.);
#18663=ADVANCED_FACE('',(#4947),#686,.T.);
#18664=ADVANCED_FACE('',(#4948),#4337,.T.);
#18665=ADVANCED_FACE('',(#4949),#4338,.T.);
#18666=ADVANCED_FACE('',(#4950),#687,.T.);
#18667=ADVANCED_FACE('',(#4951,#492),#688,.T.);
#18668=ADVANCED_FACE('',(#4952),#689,.T.);
#18669=ADVANCED_FACE('',(#4953),#690,.T.);
#18670=ADVANCED_FACE('',(#4954),#691,.T.);
#18671=ADVANCED_FACE('',(#4955),#692,.T.);
#18672=ADVANCED_FACE('',(#4956),#693,.T.);
#18673=ADVANCED_FACE('',(#4957),#694,.T.);
#18674=ADVANCED_FACE('',(#4958),#695,.T.);
#18675=ADVANCED_FACE('',(#4959,#493),#696,.T.);
#18676=ADVANCED_FACE('',(#4960,#494),#697,.T.);
#18677=ADVANCED_FACE('',(#4961,#495),#698,.T.);
#18678=ADVANCED_FACE('',(#4962,#496),#699,.T.);
#18679=ADVANCED_FACE('',(#4963,#497),#700,.T.);
#18680=ADVANCED_FACE('',(#4964,#498),#701,.T.);
#18681=ADVANCED_FACE('',(#4965,#499),#702,.T.);
#18682=ADVANCED_FACE('',(#4966,#500),#703,.T.);
#18683=ADVANCED_FACE('',(#4967),#704,.F.);
#18684=ADVANCED_FACE('',(#4968),#705,.F.);
#18685=ADVANCED_FACE('',(#4969),#706,.F.);
#18686=ADVANCED_FACE('',(#4970),#707,.F.);
#18687=ADVANCED_FACE('',(#4971),#708,.T.);
#18688=ADVANCED_FACE('',(#4972),#709,.T.);
#18689=ADVANCED_FACE('',(#4973),#710,.T.);
#18690=ADVANCED_FACE('',(#4974),#711,.T.);
#18691=ADVANCED_FACE('',(#4975),#712,.T.);
#18692=ADVANCED_FACE('',(#4976),#713,.T.);
#18693=ADVANCED_FACE('',(#4977),#714,.T.);
#18694=ADVANCED_FACE('',(#4978),#715,.F.);
#18695=ADVANCED_FACE('',(#4979),#716,.F.);
#19557=CLOSED_SHELL('',(#18555,#18556,#18557,#18558,#18559,#18560,#18561,
#18562,#18563,#18564,#18565,#18566,#18567,#18568,#18569,#18570,#18571,#18572,
#18573,#18574,#18575,#18576,#18577,#18578,#18579,#18580,#18581,#18582,#18583,
#18584,#18585,#18586,#18587,#18588,#18589,#18590,#18591,#18592,#18593,#18594,
#18595,#18596,#18597,#18598,#18599,#18600,#18601,#18602,#18603,#18604,#18605,
#18606,#18607,#18608,#18609,#18610,#18611,#18612,#18613,#18614,#18615,#18616,
#18617,#18618,#18619,#18620,#18621,#18622,#18623,#18624,#18625,#18626,#18627,
#18628,#18629,#18630,#18631,#18632,#18633,#18634,#18635,#18636,#18637,#18638,
#18639,#18640,#18641,#18642,#18643,#18644,#18645,#18646,#18647,#18648,#18649,
#18650,#18651,#18652,#18653,#18654,#18655,#18656,#18657,#18658,#18659,#18660,
#18661,#18662,#18663,#18664,#18665,#18666,#18667,#18668,#18669,#18670,#18671,
#18672,#18673,#18674,#18675,#18676,#18677,#18678,#18679,#18680,#18681,#18682,
#18683,#18684,#18685,#18686,#18687,#18688,#18689,#18690,#18691,#18692,#18693,
#18694,#18695));
#20059=AXIS2_PLACEMENT_3D('',#28721,#22536,#22537);
#20060=AXIS2_PLACEMENT_3D('',#28722,#22538,#22539);
#20061=AXIS2_PLACEMENT_3D('',#28725,#22540,#22541);
#20062=AXIS2_PLACEMENT_3D('',#28727,#22542,#22543);
#20063=AXIS2_PLACEMENT_3D('',#28729,#22544,#22545);
#20064=AXIS2_PLACEMENT_3D('',#28733,#22547,#22548);
#20065=AXIS2_PLACEMENT_3D('',#28735,#22549,#22550);
#20066=AXIS2_PLACEMENT_3D('',#28737,#22551,#22552);
#20067=AXIS2_PLACEMENT_3D('',#28781,#22556,#22557);
#20068=AXIS2_PLACEMENT_3D('',#28787,#22561,#22562);
#20069=AXIS2_PLACEMENT_3D('',#28790,#22564,#22565);
#20070=AXIS2_PLACEMENT_3D('',#28791,#22566,#22567);
#20071=AXIS2_PLACEMENT_3D('',#28794,#22569,#22570);
#20072=AXIS2_PLACEMENT_3D('',#28795,#22571,#22572);
#20073=AXIS2_PLACEMENT_3D('',#28797,#22573,#22574);
#20074=AXIS2_PLACEMENT_3D('',#28799,#22576,#22577);
#20075=AXIS2_PLACEMENT_3D('',#28803,#22580,#22581);
#20076=AXIS2_PLACEMENT_3D('',#28806,#22583,#22584);
#20077=AXIS2_PLACEMENT_3D('',#28807,#22585,#22586);
#20078=AXIS2_PLACEMENT_3D('',#28809,#22587,#22588);
#20079=AXIS2_PLACEMENT_3D('',#28810,#22589,#22590);
#20080=AXIS2_PLACEMENT_3D('',#28811,#22591,#22592);
#20081=AXIS2_PLACEMENT_3D('',#28813,#22594,#22595);
#20082=AXIS2_PLACEMENT_3D('',#28814,#22596,#22597);
#20083=AXIS2_PLACEMENT_3D('',#28820,#22601,#22602);
#20084=AXIS2_PLACEMENT_3D('',#28823,#22604,#22605);
#20085=AXIS2_PLACEMENT_3D('',#28824,#22606,#22607);
#20086=AXIS2_PLACEMENT_3D('',#28826,#22608,#22609);
#20087=AXIS2_PLACEMENT_3D('',#28828,#22611,#22612);
#20088=AXIS2_PLACEMENT_3D('',#28830,#22614,#22615);
#20089=AXIS2_PLACEMENT_3D('',#28833,#22616,#22617);
#20090=AXIS2_PLACEMENT_3D('',#28835,#22618,#22619);
#20091=AXIS2_PLACEMENT_3D('',#28837,#22620,#22621);
#20092=AXIS2_PLACEMENT_3D('',#28841,#22623,#22624);
#20093=AXIS2_PLACEMENT_3D('',#28843,#22625,#22626);
#20094=AXIS2_PLACEMENT_3D('',#28845,#22627,#22628);
#20095=AXIS2_PLACEMENT_3D('',#28889,#22632,#22633);
#20096=AXIS2_PLACEMENT_3D('',#28895,#22637,#22638);
#20097=AXIS2_PLACEMENT_3D('',#28898,#22640,#22641);
#20098=AXIS2_PLACEMENT_3D('',#28899,#22642,#22643);
#20099=AXIS2_PLACEMENT_3D('',#28902,#22645,#22646);
#20100=AXIS2_PLACEMENT_3D('',#28903,#22647,#22648);
#20101=AXIS2_PLACEMENT_3D('',#28905,#22649,#22650);
#20102=AXIS2_PLACEMENT_3D('',#28907,#22652,#22653);
#20103=AXIS2_PLACEMENT_3D('',#28911,#22656,#22657);
#20104=AXIS2_PLACEMENT_3D('',#28914,#22659,#22660);
#20105=AXIS2_PLACEMENT_3D('',#28915,#22661,#22662);
#20106=AXIS2_PLACEMENT_3D('',#28917,#22663,#22664);
#20107=AXIS2_PLACEMENT_3D('',#28918,#22665,#22666);
#20108=AXIS2_PLACEMENT_3D('',#28919,#22667,#22668);
#20109=AXIS2_PLACEMENT_3D('',#28921,#22670,#22671);
#20110=AXIS2_PLACEMENT_3D('',#28922,#22672,#22673);
#20111=AXIS2_PLACEMENT_3D('',#28928,#22677,#22678);
#20112=AXIS2_PLACEMENT_3D('',#28931,#22680,#22681);
#20113=AXIS2_PLACEMENT_3D('',#28932,#22682,#22683);
#20114=AXIS2_PLACEMENT_3D('',#28934,#22684,#22685);
#20115=AXIS2_PLACEMENT_3D('',#28936,#22687,#22688);
#20116=AXIS2_PLACEMENT_3D('',#28938,#22690,#22691);
#20117=AXIS2_PLACEMENT_3D('',#28941,#22692,#22693);
#20118=AXIS2_PLACEMENT_3D('',#28943,#22694,#22695);
#20119=AXIS2_PLACEMENT_3D('',#28945,#22696,#22697);
#20120=AXIS2_PLACEMENT_3D('',#28949,#22699,#22700);
#20121=AXIS2_PLACEMENT_3D('',#28951,#22701,#22702);
#20122=AXIS2_PLACEMENT_3D('',#28953,#22703,#22704);
#20123=AXIS2_PLACEMENT_3D('',#28997,#22708,#22709);
#20124=AXIS2_PLACEMENT_3D('',#29003,#22713,#22714);
#20125=AXIS2_PLACEMENT_3D('',#29006,#22716,#22717);
#20126=AXIS2_PLACEMENT_3D('',#29007,#22718,#22719);
#20127=AXIS2_PLACEMENT_3D('',#29010,#22721,#22722);
#20128=AXIS2_PLACEMENT_3D('',#29011,#22723,#22724);
#20129=AXIS2_PLACEMENT_3D('',#29013,#22725,#22726);
#20130=AXIS2_PLACEMENT_3D('',#29015,#22728,#22729);
#20131=AXIS2_PLACEMENT_3D('',#29019,#22732,#22733);
#20132=AXIS2_PLACEMENT_3D('',#29022,#22735,#22736);
#20133=AXIS2_PLACEMENT_3D('',#29023,#22737,#22738);
#20134=AXIS2_PLACEMENT_3D('',#29025,#22739,#22740);
#20135=AXIS2_PLACEMENT_3D('',#29026,#22741,#22742);
#20136=AXIS2_PLACEMENT_3D('',#29027,#22743,#22744);
#20137=AXIS2_PLACEMENT_3D('',#29029,#22746,#22747);
#20138=AXIS2_PLACEMENT_3D('',#29030,#22748,#22749);
#20139=AXIS2_PLACEMENT_3D('',#29036,#22753,#22754);
#20140=AXIS2_PLACEMENT_3D('',#29039,#22756,#22757);
#20141=AXIS2_PLACEMENT_3D('',#29040,#22758,#22759);
#20142=AXIS2_PLACEMENT_3D('',#29042,#22760,#22761);
#20143=AXIS2_PLACEMENT_3D('',#29044,#22763,#22764);
#20144=AXIS2_PLACEMENT_3D('',#29046,#22766,#22767);
#20145=AXIS2_PLACEMENT_3D('',#29049,#22768,#22769);
#20146=AXIS2_PLACEMENT_3D('',#29051,#22770,#22771);
#20147=AXIS2_PLACEMENT_3D('',#29053,#22772,#22773);
#20148=AXIS2_PLACEMENT_3D('',#29057,#22775,#22776);
#20149=AXIS2_PLACEMENT_3D('',#29059,#22777,#22778);
#20150=AXIS2_PLACEMENT_3D('',#29061,#22779,#22780);
#20151=AXIS2_PLACEMENT_3D('',#29105,#22784,#22785);
#20152=AXIS2_PLACEMENT_3D('',#29111,#22789,#22790);
#20153=AXIS2_PLACEMENT_3D('',#29114,#22792,#22793);
#20154=AXIS2_PLACEMENT_3D('',#29115,#22794,#22795);
#20155=AXIS2_PLACEMENT_3D('',#29118,#22797,#22798);
#20156=AXIS2_PLACEMENT_3D('',#29119,#22799,#22800);
#20157=AXIS2_PLACEMENT_3D('',#29121,#22801,#22802);
#20158=AXIS2_PLACEMENT_3D('',#29123,#22804,#22805);
#20159=AXIS2_PLACEMENT_3D('',#29127,#22808,#22809);
#20160=AXIS2_PLACEMENT_3D('',#29130,#22811,#22812);
#20161=AXIS2_PLACEMENT_3D('',#29131,#22813,#22814);
#20162=AXIS2_PLACEMENT_3D('',#29133,#22815,#22816);
#20163=AXIS2_PLACEMENT_3D('',#29134,#22817,#22818);
#20164=AXIS2_PLACEMENT_3D('',#29135,#22819,#22820);
#20165=AXIS2_PLACEMENT_3D('',#29137,#22822,#22823);
#20166=AXIS2_PLACEMENT_3D('',#29138,#22824,#22825);
#20167=AXIS2_PLACEMENT_3D('',#29144,#22829,#22830);
#20168=AXIS2_PLACEMENT_3D('',#29147,#22832,#22833);
#20169=AXIS2_PLACEMENT_3D('',#29148,#22834,#22835);
#20170=AXIS2_PLACEMENT_3D('',#29150,#22836,#22837);
#20171=AXIS2_PLACEMENT_3D('',#29152,#22839,#22840);
#20172=AXIS2_PLACEMENT_3D('',#29154,#22842,#22843);
#20173=AXIS2_PLACEMENT_3D('',#29157,#22844,#22845);
#20174=AXIS2_PLACEMENT_3D('',#29159,#22846,#22847);
#20175=AXIS2_PLACEMENT_3D('',#29161,#22848,#22849);
#20176=AXIS2_PLACEMENT_3D('',#29165,#22851,#22852);
#20177=AXIS2_PLACEMENT_3D('',#29167,#22853,#22854);
#20178=AXIS2_PLACEMENT_3D('',#29169,#22855,#22856);
#20179=AXIS2_PLACEMENT_3D('',#29213,#22860,#22861);
#20180=AXIS2_PLACEMENT_3D('',#29219,#22865,#22866);
#20181=AXIS2_PLACEMENT_3D('',#29222,#22868,#22869);
#20182=AXIS2_PLACEMENT_3D('',#29223,#22870,#22871);
#20183=AXIS2_PLACEMENT_3D('',#29226,#22873,#22874);
#20184=AXIS2_PLACEMENT_3D('',#29227,#22875,#22876);
#20185=AXIS2_PLACEMENT_3D('',#29229,#22877,#22878);
#20186=AXIS2_PLACEMENT_3D('',#29231,#22880,#22881);
#20187=AXIS2_PLACEMENT_3D('',#29235,#22884,#22885);
#20188=AXIS2_PLACEMENT_3D('',#29238,#22887,#22888);
#20189=AXIS2_PLACEMENT_3D('',#29239,#22889,#22890);
#20190=AXIS2_PLACEMENT_3D('',#29241,#22891,#22892);
#20191=AXIS2_PLACEMENT_3D('',#29242,#22893,#22894);
#20192=AXIS2_PLACEMENT_3D('',#29243,#22895,#22896);
#20193=AXIS2_PLACEMENT_3D('',#29245,#22898,#22899);
#20194=AXIS2_PLACEMENT_3D('',#29246,#22900,#22901);
#20195=AXIS2_PLACEMENT_3D('',#29252,#22905,#22906);
#20196=AXIS2_PLACEMENT_3D('',#29255,#22908,#22909);
#20197=AXIS2_PLACEMENT_3D('',#29256,#22910,#22911);
#20198=AXIS2_PLACEMENT_3D('',#29258,#22912,#22913);
#20199=AXIS2_PLACEMENT_3D('',#29260,#22915,#22916);
#20200=AXIS2_PLACEMENT_3D('',#29262,#22918,#22919);
#20201=AXIS2_PLACEMENT_3D('',#29265,#22920,#22921);
#20202=AXIS2_PLACEMENT_3D('',#29267,#22922,#22923);
#20203=AXIS2_PLACEMENT_3D('',#29269,#22924,#22925);
#20204=AXIS2_PLACEMENT_3D('',#29273,#22927,#22928);
#20205=AXIS2_PLACEMENT_3D('',#29275,#22929,#22930);
#20206=AXIS2_PLACEMENT_3D('',#29277,#22931,#22932);
#20207=AXIS2_PLACEMENT_3D('',#29321,#22936,#22937);
#20208=AXIS2_PLACEMENT_3D('',#29327,#22941,#22942);
#20209=AXIS2_PLACEMENT_3D('',#29330,#22944,#22945);
#20210=AXIS2_PLACEMENT_3D('',#29331,#22946,#22947);
#20211=AXIS2_PLACEMENT_3D('',#29334,#22949,#22950);
#20212=AXIS2_PLACEMENT_3D('',#29335,#22951,#22952);
#20213=AXIS2_PLACEMENT_3D('',#29337,#22953,#22954);
#20214=AXIS2_PLACEMENT_3D('',#29339,#22956,#22957);
#20215=AXIS2_PLACEMENT_3D('',#29343,#22960,#22961);
#20216=AXIS2_PLACEMENT_3D('',#29346,#22963,#22964);
#20217=AXIS2_PLACEMENT_3D('',#29347,#22965,#22966);
#20218=AXIS2_PLACEMENT_3D('',#29349,#22967,#22968);
#20219=AXIS2_PLACEMENT_3D('',#29350,#22969,#22970);
#20220=AXIS2_PLACEMENT_3D('',#29351,#22971,#22972);
#20221=AXIS2_PLACEMENT_3D('',#29353,#22974,#22975);
#20222=AXIS2_PLACEMENT_3D('',#29354,#22976,#22977);
#20223=AXIS2_PLACEMENT_3D('',#29360,#22981,#22982);
#20224=AXIS2_PLACEMENT_3D('',#29363,#22984,#22985);
#20225=AXIS2_PLACEMENT_3D('',#29364,#22986,#22987);
#20226=AXIS2_PLACEMENT_3D('',#29366,#22988,#22989);
#20227=AXIS2_PLACEMENT_3D('',#29368,#22991,#22992);
#20228=AXIS2_PLACEMENT_3D('',#29370,#22994,#22995);
#20229=AXIS2_PLACEMENT_3D('',#29373,#22996,#22997);
#20230=AXIS2_PLACEMENT_3D('',#29375,#22998,#22999);
#20231=AXIS2_PLACEMENT_3D('',#29377,#23000,#23001);
#20232=AXIS2_PLACEMENT_3D('',#29381,#23003,#23004);
#20233=AXIS2_PLACEMENT_3D('',#29383,#23005,#23006);
#20234=AXIS2_PLACEMENT_3D('',#29385,#23007,#23008);
#20235=AXIS2_PLACEMENT_3D('',#29429,#23012,#23013);
#20236=AXIS2_PLACEMENT_3D('',#29435,#23017,#23018);
#20237=AXIS2_PLACEMENT_3D('',#29438,#23020,#23021);
#20238=AXIS2_PLACEMENT_3D('',#29439,#23022,#23023);
#20239=AXIS2_PLACEMENT_3D('',#29442,#23025,#23026);
#20240=AXIS2_PLACEMENT_3D('',#29443,#23027,#23028);
#20241=AXIS2_PLACEMENT_3D('',#29445,#23029,#23030);
#20242=AXIS2_PLACEMENT_3D('',#29447,#23032,#23033);
#20243=AXIS2_PLACEMENT_3D('',#29451,#23036,#23037);
#20244=AXIS2_PLACEMENT_3D('',#29454,#23039,#23040);
#20245=AXIS2_PLACEMENT_3D('',#29455,#23041,#23042);
#20246=AXIS2_PLACEMENT_3D('',#29457,#23043,#23044);
#20247=AXIS2_PLACEMENT_3D('',#29458,#23045,#23046);
#20248=AXIS2_PLACEMENT_3D('',#29459,#23047,#23048);
#20249=AXIS2_PLACEMENT_3D('',#29461,#23050,#23051);
#20250=AXIS2_PLACEMENT_3D('',#29462,#23052,#23053);
#20251=AXIS2_PLACEMENT_3D('',#29468,#23057,#23058);
#20252=AXIS2_PLACEMENT_3D('',#29471,#23060,#23061);
#20253=AXIS2_PLACEMENT_3D('',#29472,#23062,#23063);
#20254=AXIS2_PLACEMENT_3D('',#29474,#23064,#23065);
#20255=AXIS2_PLACEMENT_3D('',#29476,#23067,#23068);
#20256=AXIS2_PLACEMENT_3D('',#29478,#23070,#23071);
#20257=AXIS2_PLACEMENT_3D('',#29481,#23072,#23073);
#20258=AXIS2_PLACEMENT_3D('',#29483,#23074,#23075);
#20259=AXIS2_PLACEMENT_3D('',#29485,#23076,#23077);
#20260=AXIS2_PLACEMENT_3D('',#29489,#23079,#23080);
#20261=AXIS2_PLACEMENT_3D('',#29491,#23081,#23082);
#20262=AXIS2_PLACEMENT_3D('',#29493,#23083,#23084);
#20263=AXIS2_PLACEMENT_3D('',#29537,#23088,#23089);
#20264=AXIS2_PLACEMENT_3D('',#29543,#23093,#23094);
#20265=AXIS2_PLACEMENT_3D('',#29546,#23096,#23097);
#20266=AXIS2_PLACEMENT_3D('',#29547,#23098,#23099);
#20267=AXIS2_PLACEMENT_3D('',#29550,#23101,#23102);
#20268=AXIS2_PLACEMENT_3D('',#29551,#23103,#23104);
#20269=AXIS2_PLACEMENT_3D('',#29553,#23105,#23106);
#20270=AXIS2_PLACEMENT_3D('',#29555,#23108,#23109);
#20271=AXIS2_PLACEMENT_3D('',#29559,#23112,#23113);
#20272=AXIS2_PLACEMENT_3D('',#29562,#23115,#23116);
#20273=AXIS2_PLACEMENT_3D('',#29563,#23117,#23118);
#20274=AXIS2_PLACEMENT_3D('',#29565,#23119,#23120);
#20275=AXIS2_PLACEMENT_3D('',#29566,#23121,#23122);
#20276=AXIS2_PLACEMENT_3D('',#29567,#23123,#23124);
#20277=AXIS2_PLACEMENT_3D('',#29569,#23126,#23127);
#20278=AXIS2_PLACEMENT_3D('',#29570,#23128,#23129);
#20279=AXIS2_PLACEMENT_3D('',#29576,#23133,#23134);
#20280=AXIS2_PLACEMENT_3D('',#29579,#23136,#23137);
#20281=AXIS2_PLACEMENT_3D('',#29580,#23138,#23139);
#20282=AXIS2_PLACEMENT_3D('',#29582,#23140,#23141);
#20283=AXIS2_PLACEMENT_3D('',#29584,#23142,#23143);
#20284=AXIS2_PLACEMENT_3D('',#29586,#23144,#23145);
#20285=AXIS2_PLACEMENT_3D('',#29588,#23147,#23148);
#20286=AXIS2_PLACEMENT_3D('',#29590,#23150,#23151);
#20287=AXIS2_PLACEMENT_3D('',#29623,#23168,#23169);
#20288=AXIS2_PLACEMENT_3D('',#29629,#23173,#23174);
#20289=AXIS2_PLACEMENT_3D('',#29633,#23177,#23178);
#20290=AXIS2_PLACEMENT_3D('',#29639,#23182,#23183);
#20291=AXIS2_PLACEMENT_3D('',#29647,#23188,#23189);
#20292=AXIS2_PLACEMENT_3D('',#29651,#23192,#23193);
#20293=AXIS2_PLACEMENT_3D('',#29655,#23196,#23197);
#20294=AXIS2_PLACEMENT_3D('',#29657,#23199,#23200);
#20295=AXIS2_PLACEMENT_3D('',#29687,#23216,#23217);
#20296=AXIS2_PLACEMENT_3D('',#29690,#23220,#23221);
#20297=AXIS2_PLACEMENT_3D('',#29692,#23223,#23224);
#20298=AXIS2_PLACEMENT_3D('',#29694,#23226,#23227);
#20299=AXIS2_PLACEMENT_3D('',#29696,#23229,#23230);
#20300=AXIS2_PLACEMENT_3D('',#29698,#23232,#23233);
#20301=AXIS2_PLACEMENT_3D('',#29700,#23235,#23236);
#20302=AXIS2_PLACEMENT_3D('',#29702,#23238,#23239);
#20303=AXIS2_PLACEMENT_3D('',#29713,#23246,#23247);
#20304=AXIS2_PLACEMENT_3D('',#29722,#23253,#23254);
#20305=AXIS2_PLACEMENT_3D('',#29731,#23260,#23261);
#20306=AXIS2_PLACEMENT_3D('',#29732,#23262,#23263);
#20307=AXIS2_PLACEMENT_3D('',#29740,#23269,#23270);
#20308=AXIS2_PLACEMENT_3D('',#29743,#23273,#23274);
#20309=AXIS2_PLACEMENT_3D('',#29746,#23277,#23278);
#20310=AXIS2_PLACEMENT_3D('',#29747,#23279,#23280);
#20311=AXIS2_PLACEMENT_3D('',#29748,#23281,#23282);
#20312=AXIS2_PLACEMENT_3D('',#29749,#23283,#23284);
#20313=AXIS2_PLACEMENT_3D('',#29750,#23285,#23286);
#20314=AXIS2_PLACEMENT_3D('',#29752,#23288,#23289);
#22536=DIRECTION('axis',(0.,0.,1.));
#22537=DIRECTION('refdir',(1.,0.,0.));
#22538=DIRECTION('center_axis',(0.,-1.,0.));
#22539=DIRECTION('ref_axis',(1.,0.,0.));
#22540=DIRECTION('center_axis',(0.3582068848149,-0.554700196225404,0.75099635150825));
#22541=DIRECTION('ref_axis',(0.238804589876937,0.832050294337727,0.500664234338952));
#22542=DIRECTION('center_axis',(0.,1.,0.));
#22543=DIRECTION('ref_axis',(1.,0.,0.));
#22544=DIRECTION('center_axis',(-0.75099635150825,-0.554700196225404,-0.3582068848149));
#22545=DIRECTION('ref_axis',(0.500664234338953,-0.832050294337727,0.238804589876937));
#22546=DIRECTION('',(0.,1.,0.));
#22547=DIRECTION('center_axis',(-0.75099635150825,0.554700196225404,-0.3582068848149));
#22548=DIRECTION('ref_axis',(0.500664234338953,0.832050294337727,0.238804589876937));
#22549=DIRECTION('center_axis',(0.,1.,0.));
#22550=DIRECTION('ref_axis',(1.,0.,0.));
#22551=DIRECTION('center_axis',(0.3582068848149,0.554700196225404,0.75099635150825));
#22552=DIRECTION('ref_axis',(0.238804589876937,-0.832050294337727,0.500664234338952));
#22553=DIRECTION('',(0.,-1.,0.));
#22554=DIRECTION('',(0.,1.,0.));
#22555=DIRECTION('',(0.,-1.,0.));
#22556=DIRECTION('center_axis',(-0.430511096808295,0.,-0.902585284349861));
#22557=DIRECTION('ref_axis',(-0.902585284349861,0.,0.430511096808295));
#22558=DIRECTION('',(-0.902585284349657,0.,0.430511096808721));
#22559=DIRECTION('',(0.902585284349657,0.,-0.430511096808721));
#22560=DIRECTION('',(0.,1.,0.));
#22561=DIRECTION('center_axis',(0.35820688481505,0.554700196225229,0.750996351508308));
#22562=DIRECTION('ref_axis',(0.84006490861712,-0.542485897798375,-2.44189949696171E-17));
#22563=DIRECTION('',(-0.902585284349657,0.,0.430511096808721));
#22564=DIRECTION('center_axis',(-0.358206884814892,-0.554700196225413,-0.750996351508247));
#22565=DIRECTION('ref_axis',(-0.238804589876949,0.832050294337721,-0.500664234338957));
#22566=DIRECTION('center_axis',(0.,1.,0.));
#22567=DIRECTION('ref_axis',(1.,0.,0.));
#22568=DIRECTION('',(0.430511096808721,0.,-0.902585284349657));
#22569=DIRECTION('center_axis',(0.,-1.,0.));
#22570=DIRECTION('ref_axis',(-1.,0.,0.));
#22571=DIRECTION('center_axis',(-0.750996351508308,0.554700196225229,-0.35820688481505));
#22572=DIRECTION('ref_axis',(-0.430511096808295,9.35899339744592E-17,0.902585284349861));
#22573=DIRECTION('center_axis',(0.750996351508247,-0.554700196225414,0.358206884814892));
#22574=DIRECTION('ref_axis',(-0.500664234338957,-0.83205029433772,-0.23880458987695));
#22575=DIRECTION('',(-0.430511096808721,0.,0.902585284349657));
#22576=DIRECTION('center_axis',(0.902585284349861,0.,0.430511096808295));
#22577=DIRECTION('ref_axis',(0.,-1.,0.));
#22578=DIRECTION('',(0.430511096808721,0.,-0.902585284349657));
#22579=DIRECTION('',(0.,-1.,0.));
#22580=DIRECTION('center_axis',(-0.750996351508308,-0.554700196225229,-0.35820688481505));
#22581=DIRECTION('ref_axis',(-0.594125001994256,0.804372725796521,-4.34111046316595E-17));
#22582=DIRECTION('',(-0.430511096808721,0.,0.902585284349657));
#22583=DIRECTION('center_axis',(0.750996351508247,0.554700196225413,0.358206884814892));
#22584=DIRECTION('ref_axis',(-0.500664234338957,0.832050294337721,-0.238804589876949));
#22585=DIRECTION('center_axis',(0.,-1.,0.));
#22586=DIRECTION('ref_axis',(-1.,0.,0.));
#22587=DIRECTION('center_axis',(-0.358206884814892,0.554700196225413,-0.750996351508247));
#22588=DIRECTION('ref_axis',(-0.238804589876949,-0.832050294337721,-0.500664234338957));
#22589=DIRECTION('center_axis',(0.,-1.,0.));
#22590=DIRECTION('ref_axis',(-1.,0.,0.));
#22591=DIRECTION('center_axis',(0.,-1.,0.));
#22592=DIRECTION('ref_axis',(0.,0.,-1.));
#22593=DIRECTION('',(0.902585284349657,0.,-0.430511096808721));
#22594=DIRECTION('center_axis',(0.35820688481505,-0.554700196225229,0.750996351508308));
#22595=DIRECTION('ref_axis',(-0.84006490861712,-0.542485897798375,2.44189949696171E-17));
#22596=DIRECTION('center_axis',(-0.707106781186548,1.63268091856641E-16,
-0.707106781186548));
#22597=DIRECTION('ref_axis',(-0.707106781186548,1.6035606412684E-33,0.707106781186548));
#22598=DIRECTION('',(-0.707106781186548,0.,0.707106781186548));
#22599=DIRECTION('',(-1.0001154479739E-12,-1.,-1.0001154479739E-12));
#22600=DIRECTION('',(-0.707106781186548,0.,0.707106781186548));
#22601=DIRECTION('center_axis',(-0.707106781186548,0.,0.707106781186548));
#22602=DIRECTION('ref_axis',(0.707106781186547,0.,0.707106781186547));
#22603=DIRECTION('',(-0.707106781186548,0.,0.707106781186548));
#22604=DIRECTION('center_axis',(-0.707106781186548,0.,0.707106781186548));
#22605=DIRECTION('ref_axis',(0.707106781186547,0.,0.707106781186547));
#22606=DIRECTION('center_axis',(-0.707106781186548,0.,0.707106781186548));
#22607=DIRECTION('ref_axis',(-0.707106781186547,0.,-0.707106781186547));
#22608=DIRECTION('center_axis',(-0.707106781186548,0.,0.707106781186548));
#22609=DIRECTION('ref_axis',(-0.707106781186547,0.,-0.707106781186547));
#22610=DIRECTION('',(-0.707106781186548,0.,0.707106781186548));
#22611=DIRECTION('center_axis',(0.707106781186548,8.16340459283203E-17,
0.707106781186548));
#22612=DIRECTION('ref_axis',(-1.81589014284111E-31,-1.,1.15447974903219E-16));
#22613=DIRECTION('',(-1.00005772398645E-12,1.,-1.00005772398645E-12));
#22614=DIRECTION('center_axis',(0.,-1.,0.));
#22615=DIRECTION('ref_axis',(0.707106781186548,0.,-0.707106781186548));
#22616=DIRECTION('center_axis',(0.784325130117969,-0.554700196225389,0.277744095478098));
#22617=DIRECTION('ref_axis',(0.522883420078948,0.832050294337737,0.185162730318571));
#22618=DIRECTION('center_axis',(0.,1.,0.));
#22619=DIRECTION('ref_axis',(0.707106781186547,0.,-0.707106781186547));
#22620=DIRECTION('center_axis',(-0.784325130117969,-0.554700196225389,0.277744095478098));
#22621=DIRECTION('ref_axis',(0.522883420078948,-0.832050294337737,-0.185162730318571));
#22622=DIRECTION('',(0.,1.,0.));
#22623=DIRECTION('center_axis',(-0.784325130117969,0.554700196225389,0.277744095478098));
#22624=DIRECTION('ref_axis',(0.522883420078948,0.832050294337737,-0.185162730318571));
#22625=DIRECTION('center_axis',(0.,1.,0.));
#22626=DIRECTION('ref_axis',(0.707106781186547,0.,-0.707106781186547));
#22627=DIRECTION('center_axis',(0.784325130117969,0.554700196225389,0.277744095478098));
#22628=DIRECTION('ref_axis',(0.522883420078948,-0.832050294337737,0.185162730318571));
#22629=DIRECTION('',(0.,-1.,0.));
#22630=DIRECTION('',(0.,1.,0.));
#22631=DIRECTION('',(0.,-1.,0.));
#22632=DIRECTION('center_axis',(-0.942641491092178,0.,-0.333806859233771));
#22633=DIRECTION('ref_axis',(-0.333806859233771,0.,0.942641491092178));
#22634=DIRECTION('',(-0.333806859234345,0.,0.942641491091975));
#22635=DIRECTION('',(0.333806859234345,0.,-0.942641491091975));
#22636=DIRECTION('',(0.,1.,0.));
#22637=DIRECTION('center_axis',(0.784325130118311,0.554700196225229,0.27774409547745));
#22638=DIRECTION('ref_axis',(1.41728662356081E-16,0.447721620230319,-0.894172998238226));
#22639=DIRECTION('',(-0.333806859234345,0.,0.942641491091975));
#22640=DIRECTION('center_axis',(-0.78432513011795,-0.554700196225397,-0.277744095478133));
#22641=DIRECTION('ref_axis',(-0.522883420078951,0.832050294337732,-0.185162730318585));
#22642=DIRECTION('center_axis',(0.,1.,0.));
#22643=DIRECTION('ref_axis',(1.,0.,0.));
#22644=DIRECTION('',(-0.333806859234345,0.,-0.942641491091975));
#22645=DIRECTION('center_axis',(0.,-1.,0.));
#22646=DIRECTION('ref_axis',(-0.707106781186548,0.,0.707106781186548));
#22647=DIRECTION('center_axis',(-0.784325130118311,0.554700196225229,0.27774409547745));
#22648=DIRECTION('ref_axis',(0.333806859233771,9.47580827855939E-17,0.942641491092179));
#22649=DIRECTION('center_axis',(0.78432513011795,-0.554700196225398,-0.277744095478132));
#22650=DIRECTION('ref_axis',(-0.522883420078952,-0.832050294337731,0.185162730318585));
#22651=DIRECTION('',(0.333806859234345,0.,0.942641491091975));
#22652=DIRECTION('center_axis',(0.942641491092178,0.,-0.333806859233771));
#22653=DIRECTION('ref_axis',(0.,-1.,0.));
#22654=DIRECTION('',(-0.333806859234345,0.,-0.942641491091975));
#22655=DIRECTION('',(0.,-1.,0.));
#22656=DIRECTION('center_axis',(-0.784325130118311,-0.554700196225229,0.27774409547745));
#22657=DIRECTION('ref_axis',(-0.577418677468947,0.816448204670702,-1.57337619069903E-16));
#22658=DIRECTION('',(0.333806859234345,0.,0.942641491091975));
#22659=DIRECTION('center_axis',(0.78432513011795,0.554700196225397,-0.277744095478133));
#22660=DIRECTION('ref_axis',(-0.522883420078951,0.832050294337732,0.185162730318585));
#22661=DIRECTION('center_axis',(0.,-1.,0.));
#22662=DIRECTION('ref_axis',(-0.707106781186548,0.,0.707106781186548));
#22663=DIRECTION('center_axis',(-0.78432513011795,0.554700196225397,-0.277744095478133));
#22664=DIRECTION('ref_axis',(-0.522883420078951,-0.832050294337732,-0.185162730318585));
#22665=DIRECTION('center_axis',(0.,-1.,0.));
#22666=DIRECTION('ref_axis',(-0.707106781186548,0.,0.707106781186548));
#22667=DIRECTION('center_axis',(0.,-1.,0.));
#22668=DIRECTION('ref_axis',(0.,0.,-1.));
#22669=DIRECTION('',(0.333806859234345,0.,-0.942641491091975));
#22670=DIRECTION('center_axis',(0.784325130118311,-0.554700196225229,0.27774409547745));
#22671=DIRECTION('ref_axis',(1.41728662356081E-16,-0.447721620230319,-0.894172998238226));
#22672=DIRECTION('center_axis',(-1.,1.63268091856641E-16,0.));
#22673=DIRECTION('ref_axis',(0.,0.,1.));
#22674=DIRECTION('',(0.,0.,1.));
#22675=DIRECTION('',(-1.00016326809086E-12,-1.,0.));
#22676=DIRECTION('',(0.,0.,1.));
#22677=DIRECTION('center_axis',(0.,0.,1.));
#22678=DIRECTION('ref_axis',(1.,0.,0.));
#22679=DIRECTION('',(0.,0.,1.));
#22680=DIRECTION('center_axis',(0.,0.,1.));
#22681=DIRECTION('ref_axis',(1.,0.,0.));
#22682=DIRECTION('center_axis',(0.,0.,1.));
#22683=DIRECTION('ref_axis',(-1.,0.,0.));
#22684=DIRECTION('center_axis',(0.,0.,1.));
#22685=DIRECTION('ref_axis',(-1.,0.,0.));
#22686=DIRECTION('',(0.,0.,1.));
#22687=DIRECTION('center_axis',(1.,5.4401887036275E-49,6.66411745462711E-33));
#22688=DIRECTION('ref_axis',(4.75910974851396E-64,1.,-8.16340459283203E-17));
#22689=DIRECTION('',(-1.00008163404493E-12,1.,0.));
#22690=DIRECTION('center_axis',(0.,-1.,0.));
#22691=DIRECTION('ref_axis',(0.,0.,-1.));
#22692=DIRECTION('center_axis',(0.75099635150825,-0.554700196225404,-0.3582068848149));
#22693=DIRECTION('ref_axis',(0.500664234338953,0.832050294337727,-0.238804589876937));
#22694=DIRECTION('center_axis',(0.,1.,0.));
#22695=DIRECTION('ref_axis',(0.,0.,-1.));
#22696=DIRECTION('center_axis',(-0.3582068848149,-0.554700196225404,0.75099635150825));
#22697=DIRECTION('ref_axis',(0.238804589876937,-0.832050294337727,-0.500664234338952));
#22698=DIRECTION('',(0.,1.,0.));
#22699=DIRECTION('center_axis',(-0.3582068848149,0.554700196225404,0.75099635150825));
#22700=DIRECTION('ref_axis',(0.238804589876937,0.832050294337727,-0.500664234338953));
#22701=DIRECTION('center_axis',(0.,1.,0.));
#22702=DIRECTION('ref_axis',(0.,0.,-1.));
#22703=DIRECTION('center_axis',(0.75099635150825,0.554700196225404,-0.3582068848149));
#22704=DIRECTION('ref_axis',(0.500664234338953,-0.832050294337727,-0.238804589876937));
#22705=DIRECTION('',(0.,-1.,0.));
#22706=DIRECTION('',(0.,1.,0.));
#22707=DIRECTION('',(0.,-1.,0.));
#22708=DIRECTION('center_axis',(-0.902585284349861,0.,0.430511096808295));
#22709=DIRECTION('ref_axis',(0.,1.,0.));
#22710=DIRECTION('',(0.430511096808721,0.,0.902585284349657));
#22711=DIRECTION('',(-0.430511096808721,0.,-0.902585284349657));
#22712=DIRECTION('',(0.,1.,0.));
#22713=DIRECTION('center_axis',(0.750996351508308,0.554700196225229,-0.35820688481505));
#22714=DIRECTION('ref_axis',(-2.67556946657892E-17,-0.542485897798375,-0.84006490861712));
#22715=DIRECTION('',(0.430511096808721,0.,0.902585284349657));
#22716=DIRECTION('center_axis',(-0.750996351508247,-0.554700196225413,0.358206884814892));
#22717=DIRECTION('ref_axis',(-0.500664234338957,0.832050294337721,0.238804589876949));
#22718=DIRECTION('center_axis',(0.,1.,0.));
#22719=DIRECTION('ref_axis',(1.,0.,0.));
#22720=DIRECTION('',(-0.902585284349657,0.,-0.430511096808721));
#22721=DIRECTION('center_axis',(0.,-1.,0.));
#22722=DIRECTION('ref_axis',(0.,0.,1.));
#22723=DIRECTION('center_axis',(-0.35820688481505,0.554700196225229,0.750996351508308));
#22724=DIRECTION('ref_axis',(0.84006490861712,0.542485897798375,2.44189949696171E-17));
#22725=DIRECTION('center_axis',(0.358206884814892,-0.554700196225414,-0.750996351508247));
#22726=DIRECTION('ref_axis',(-0.23880458987695,-0.83205029433772,0.500664234338957));
#22727=DIRECTION('',(0.902585284349657,0.,0.430511096808721));
#22728=DIRECTION('center_axis',(0.430511096808295,0.,-0.902585284349861));
#22729=DIRECTION('ref_axis',(0.,-1.,0.));
#22730=DIRECTION('',(-0.902585284349657,0.,-0.430511096808721));
#22731=DIRECTION('',(0.,-1.,0.));
#22732=DIRECTION('center_axis',(-0.35820688481505,-0.554700196225229,0.750996351508308));
#22733=DIRECTION('ref_axis',(-0.84006490861712,0.542485897798375,-2.44189949696171E-17));
#22734=DIRECTION('',(0.902585284349657,0.,0.430511096808721));
#22735=DIRECTION('center_axis',(0.358206884814892,0.554700196225413,-0.750996351508247));
#22736=DIRECTION('ref_axis',(-0.238804589876949,0.832050294337721,0.500664234338957));
#22737=DIRECTION('center_axis',(0.,-1.,0.));
#22738=DIRECTION('ref_axis',(0.,0.,1.));
#22739=DIRECTION('center_axis',(-0.750996351508247,0.554700196225413,0.358206884814892));
#22740=DIRECTION('ref_axis',(-0.500664234338957,-0.832050294337721,0.238804589876949));
#22741=DIRECTION('center_axis',(0.,-1.,0.));
#22742=DIRECTION('ref_axis',(0.,0.,1.));
#22743=DIRECTION('center_axis',(0.,-1.,0.));
#22744=DIRECTION('ref_axis',(0.,0.,-1.));
#22745=DIRECTION('',(-0.430511096808721,0.,-0.902585284349657));
#22746=DIRECTION('center_axis',(0.750996351508308,-0.554700196225229,-0.35820688481505));
#22747=DIRECTION('ref_axis',(-2.67556946657892E-17,0.542485897798375,-0.84006490861712));
#22748=DIRECTION('center_axis',(-0.707106781186548,1.63268091856641E-16,
0.707106781186548));
#22749=DIRECTION('ref_axis',(2.30895949806438E-16,1.,9.37581606751804E-32));
#22750=DIRECTION('',(0.707106781186548,0.,0.707106781186548));
#22751=DIRECTION('',(-1.0001154479739E-12,-1.,1.0001154479739E-12));
#22752=DIRECTION('',(0.707106781186548,0.,0.707106781186548));
#22753=DIRECTION('center_axis',(0.707106781186548,0.,0.707106781186548));
#22754=DIRECTION('ref_axis',(0.707106781186547,0.,-0.707106781186547));
#22755=DIRECTION('',(0.707106781186548,0.,0.707106781186548));
#22756=DIRECTION('center_axis',(0.707106781186548,0.,0.707106781186548));
#22757=DIRECTION('ref_axis',(0.707106781186547,0.,-0.707106781186547));
#22758=DIRECTION('center_axis',(0.707106781186548,0.,0.707106781186548));
#22759=DIRECTION('ref_axis',(-0.707106781186547,0.,0.707106781186547));
#22760=DIRECTION('center_axis',(0.707106781186548,0.,0.707106781186548));
#22761=DIRECTION('ref_axis',(-0.707106781186547,0.,0.707106781186547));
#22762=DIRECTION('',(0.707106781186548,0.,0.707106781186548));
#22763=DIRECTION('center_axis',(0.707106781186548,8.16340459283203E-17,
-0.707106781186548));
#22764=DIRECTION('ref_axis',(-1.81589014284111E-31,-1.,-1.15447974903219E-16));
#22765=DIRECTION('',(-1.00005772398645E-12,1.,1.00005772398645E-12));
#22766=DIRECTION('center_axis',(0.,-1.,0.));
#22767=DIRECTION('ref_axis',(-0.707106781186547,0.,-0.707106781186548));
#22768=DIRECTION('center_axis',(0.277744095478098,-0.554700196225389,-0.784325130117969));
#22769=DIRECTION('ref_axis',(0.185162730318571,0.832050294337737,-0.522883420078948));
#22770=DIRECTION('center_axis',(0.,1.,0.));
#22771=DIRECTION('ref_axis',(-0.707106781186547,0.,-0.707106781186548));
#22772=DIRECTION('center_axis',(0.277744095478098,-0.554700196225389,0.784325130117969));
#22773=DIRECTION('ref_axis',(-0.185162730318571,-0.832050294337737,-0.522883420078948));
#22774=DIRECTION('',(0.,1.,0.));
#22775=DIRECTION('center_axis',(0.277744095478098,0.554700196225389,0.784325130117969));
#22776=DIRECTION('ref_axis',(-0.185162730318571,0.832050294337737,-0.522883420078948));
#22777=DIRECTION('center_axis',(0.,1.,0.));
#22778=DIRECTION('ref_axis',(-0.707106781186547,0.,-0.707106781186548));
#22779=DIRECTION('center_axis',(0.277744095478098,0.554700196225389,-0.784325130117969));
#22780=DIRECTION('ref_axis',(0.185162730318571,-0.832050294337737,-0.522883420078948));
#22781=DIRECTION('',(0.,-1.,0.));
#22782=DIRECTION('',(0.,1.,0.));
#22783=DIRECTION('',(0.,-1.,0.));
#22784=DIRECTION('center_axis',(-0.333806859233771,0.,0.942641491092178));
#22785=DIRECTION('ref_axis',(0.,1.,0.));
#22786=DIRECTION('',(0.942641491091975,0.,0.333806859234345));
#22787=DIRECTION('',(-0.942641491091975,0.,-0.333806859234345));
#22788=DIRECTION('',(0.,1.,0.));
#22789=DIRECTION('center_axis',(0.27774409547745,0.554700196225229,-0.784325130118311));
#22790=DIRECTION('ref_axis',(-0.942641491092179,-8.22449654774124E-17,-0.333806859233771));
#22791=DIRECTION('',(0.942641491091975,0.,0.333806859234345));
#22792=DIRECTION('center_axis',(-0.277744095478133,-0.554700196225397,0.78432513011795));
#22793=DIRECTION('ref_axis',(-0.185162730318585,0.832050294337732,0.522883420078951));
#22794=DIRECTION('center_axis',(0.,1.,0.));
#22795=DIRECTION('ref_axis',(1.,0.,0.));
#22796=DIRECTION('',(-0.942641491091975,0.,0.333806859234345));
#22797=DIRECTION('center_axis',(0.,-1.,0.));
#22798=DIRECTION('ref_axis',(0.707106781186547,0.,0.707106781186548));
#22799=DIRECTION('center_axis',(0.27774409547745,0.554700196225229,0.784325130118311));
#22800=DIRECTION('ref_axis',(0.894172998238226,-0.447721620230319,-1.29766088156978E-16));
#22801=DIRECTION('center_axis',(-0.277744095478132,-0.554700196225398,-0.78432513011795));
#22802=DIRECTION('ref_axis',(0.185162730318585,-0.832050294337731,0.522883420078952));
#22803=DIRECTION('',(0.942641491091975,0.,-0.333806859234345));
#22804=DIRECTION('center_axis',(-0.333806859233771,0.,-0.942641491092178));
#22805=DIRECTION('ref_axis',(-0.942641491092178,0.,0.333806859233771));
#22806=DIRECTION('',(-0.942641491091975,0.,0.333806859234345));
#22807=DIRECTION('',(0.,-1.,0.));
#22808=DIRECTION('center_axis',(0.27774409547745,-0.554700196225229,0.784325130118311));
#22809=DIRECTION('ref_axis',(-0.894172998238226,-0.447721620230319,1.29766088156978E-16));
#22810=DIRECTION('',(0.942641491091975,0.,-0.333806859234345));
#22811=DIRECTION('center_axis',(-0.277744095478133,0.554700196225397,-0.78432513011795));
#22812=DIRECTION('ref_axis',(0.185162730318585,0.832050294337732,0.522883420078951));
#22813=DIRECTION('center_axis',(0.,-1.,0.));
#22814=DIRECTION('ref_axis',(0.707106781186547,0.,0.707106781186548));
#22815=DIRECTION('center_axis',(-0.277744095478133,0.554700196225397,0.78432513011795));
#22816=DIRECTION('ref_axis',(-0.185162730318585,-0.832050294337732,0.522883420078951));
#22817=DIRECTION('center_axis',(0.,-1.,0.));
#22818=DIRECTION('ref_axis',(0.707106781186547,0.,0.707106781186548));
#22819=DIRECTION('center_axis',(0.,-1.,0.));
#22820=DIRECTION('ref_axis',(0.,0.,-1.));
#22821=DIRECTION('',(-0.942641491091975,0.,-0.333806859234345));
#22822=DIRECTION('center_axis',(0.27774409547745,-0.554700196225229,-0.784325130118311));
#22823=DIRECTION('ref_axis',(1.53589745588664E-16,-0.816448204670702,0.577418677468947));
#22824=DIRECTION('center_axis',(-1.81263994765859E-32,1.63268091856641E-16,
1.));
#22825=DIRECTION('ref_axis',(1.,1.11022302462516E-16,5.86020957047602E-47));
#22826=DIRECTION('',(1.,0.,1.00011102230146E-12));
#22827=DIRECTION('',(-9.99999999999E-13,-1.,1.00016326809086E-12));
#22828=DIRECTION('',(1.,0.,1.00011102230146E-12));
#22829=DIRECTION('center_axis',(1.,0.,1.85037170770859E-16));
#22830=DIRECTION('ref_axis',(1.85037170770859E-16,0.,-1.));
#22831=DIRECTION('',(1.,0.,1.00011102230146E-12));
#22832=DIRECTION('center_axis',(1.,0.,6.66685170379299E-12));
#22833=DIRECTION('ref_axis',(6.66685170379299E-12,0.,-1.));
#22834=DIRECTION('center_axis',(1.,0.,9.25185853854296E-17));
#22835=DIRECTION('ref_axis',(-9.25185853854296E-17,0.,1.));
#22836=DIRECTION('center_axis',(1.,0.,6.66675918520761E-12));
#22837=DIRECTION('ref_axis',(-6.66675918520761E-12,0.,1.));
#22838=DIRECTION('',(1.,0.,1.00011102230146E-12));
#22839=DIRECTION('center_axis',(1.11022302462516E-16,8.16340459283203E-17,
-1.));
#22840=DIRECTION('ref_axis',(0.,-1.,-8.16340459283203E-17));
#22841=DIRECTION('',(-9.99999999999E-13,1.,1.00008163404493E-12));
#22842=DIRECTION('center_axis',(0.,-1.,0.));
#22843=DIRECTION('ref_axis',(-1.,0.,-1.51566283225277E-16));
#22844=DIRECTION('center_axis',(-0.3582068848149,-0.554700196225404,-0.75099635150825));
#22845=DIRECTION('ref_axis',(-0.238804589876937,0.832050294337727,-0.500664234338952));
#22846=DIRECTION('center_axis',(0.,1.,0.));
#22847=DIRECTION('ref_axis',(-1.,0.,-6.82745422938049E-13));
#22848=DIRECTION('center_axis',(0.75099635150825,-0.554700196225404,0.3582068848149));
#22849=DIRECTION('ref_axis',(-0.500664234338953,-0.832050294337727,-0.238804589876937));
#22850=DIRECTION('',(0.,1.,0.));
#22851=DIRECTION('center_axis',(0.75099635150825,0.554700196225404,0.3582068848149));
#22852=DIRECTION('ref_axis',(-0.500664234338953,0.832050294337727,-0.238804589876937));
#22853=DIRECTION('center_axis',(0.,1.,0.));
#22854=DIRECTION('ref_axis',(-1.,0.,-6.82745422938049E-13));
#22855=DIRECTION('center_axis',(-0.3582068848149,0.554700196225404,-0.75099635150825));
#22856=DIRECTION('ref_axis',(-0.238804589876937,-0.832050294337727,-0.500664234338952));
#22857=DIRECTION('',(0.,-1.,0.));
#22858=DIRECTION('',(0.,1.,0.));
#22859=DIRECTION('',(0.,-1.,0.));
#22860=DIRECTION('center_axis',(0.430511096808295,0.,0.902585284349861));
#22861=DIRECTION('ref_axis',(0.,-1.,0.));
#22862=DIRECTION('',(0.902585284349657,0.,-0.430511096808721));
#22863=DIRECTION('',(-0.902585284349657,0.,0.430511096808721));
#22864=DIRECTION('',(0.,1.,0.));
#22865=DIRECTION('center_axis',(-0.35820688481505,0.554700196225229,-0.750996351508308));
#22866=DIRECTION('ref_axis',(-0.902585284349861,-8.75902672829316E-17,0.430511096808295));
#22867=DIRECTION('',(0.902585284349657,0.,-0.430511096808721));
#22868=DIRECTION('center_axis',(0.358206884814892,-0.554700196225413,0.750996351508247));
#22869=DIRECTION('ref_axis',(0.238804589876949,0.832050294337721,0.500664234338957));
#22870=DIRECTION('center_axis',(0.,1.,0.));
#22871=DIRECTION('ref_axis',(1.,0.,0.));
#22872=DIRECTION('',(-0.430511096808721,0.,0.902585284349657));
#22873=DIRECTION('center_axis',(0.,-1.,0.));
#22874=DIRECTION('ref_axis',(1.,0.,7.19584204751227E-13));
#22875=DIRECTION('center_axis',(0.750996351508308,0.554700196225229,0.35820688481505));
#22876=DIRECTION('ref_axis',(2.67556946657892E-17,0.542485897798375,-0.84006490861712));
#22877=DIRECTION('center_axis',(-0.750996351508247,-0.554700196225414,-0.358206884814892));
#22878=DIRECTION('ref_axis',(0.500664234338957,-0.83205029433772,0.23880458987695));
#22879=DIRECTION('',(0.430511096808721,0.,-0.902585284349657));
#22880=DIRECTION('center_axis',(-0.902585284349861,0.,-0.430511096808295));
#22881=DIRECTION('ref_axis',(-0.430511096808295,0.,0.902585284349861));
#22882=DIRECTION('',(-0.430511096808721,0.,0.902585284349657));
#22883=DIRECTION('',(0.,-1.,0.));
#22884=DIRECTION('center_axis',(0.750996351508308,-0.554700196225229,0.35820688481505));
#22885=DIRECTION('ref_axis',(2.67556946657892E-17,-0.542485897798375,-0.84006490861712));
#22886=DIRECTION('',(0.430511096808721,0.,-0.902585284349657));
#22887=DIRECTION('center_axis',(-0.750996351508247,0.554700196225413,-0.358206884814892));
#22888=DIRECTION('ref_axis',(0.500664234338957,0.832050294337721,0.238804589876949));
#22889=DIRECTION('center_axis',(0.,-1.,0.));
#22890=DIRECTION('ref_axis',(1.,0.,1.59744320089951E-16));
#22891=DIRECTION('center_axis',(0.358206884814892,0.554700196225413,0.750996351508247));
#22892=DIRECTION('ref_axis',(0.238804589876949,-0.832050294337721,0.500664234338957));
#22893=DIRECTION('center_axis',(0.,-1.,0.));
#22894=DIRECTION('ref_axis',(1.,0.,7.19584204751227E-13));
#22895=DIRECTION('center_axis',(0.,-1.,0.));
#22896=DIRECTION('ref_axis',(0.,0.,-1.));
#22897=DIRECTION('',(-0.902585284349657,0.,0.430511096808721));
#22898=DIRECTION('center_axis',(-0.35820688481505,-0.554700196225229,-0.750996351508308));
#22899=DIRECTION('ref_axis',(4.41754862127715E-17,-0.804372725796521,0.594125001994256));
#22900=DIRECTION('center_axis',(0.707106781186547,1.63268091856641E-16,
0.707106781186548));
#22901=DIRECTION('ref_axis',(2.30895949806438E-16,-1.,7.31254524561613E-32));
#22902=DIRECTION('',(0.707106781186548,0.,-0.707106781186547));
#22903=DIRECTION('',(1.0001154479739E-12,-1.,1.0001154479739E-12));
#22904=DIRECTION('',(0.707106781186548,0.,-0.707106781186547));
#22905=DIRECTION('center_axis',(0.707106781186548,0.,-0.707106781186547));
#22906=DIRECTION('ref_axis',(-0.707106781186547,0.,-0.707106781186548));
#22907=DIRECTION('',(0.707106781186548,0.,-0.707106781186547));
#22908=DIRECTION('center_axis',(0.707106781186548,0.,-0.707106781186547));
#22909=DIRECTION('ref_axis',(-0.707106781186547,0.,-0.707106781186548));
#22910=DIRECTION('center_axis',(0.707106781186548,0.,-0.707106781186547));
#22911=DIRECTION('ref_axis',(0.707106781186547,0.,0.707106781186548));
#22912=DIRECTION('center_axis',(0.707106781186548,0.,-0.707106781186547));
#22913=DIRECTION('ref_axis',(0.707106781186547,0.,0.707106781186548));
#22914=DIRECTION('',(0.707106781186548,0.,-0.707106781186547));
#22915=DIRECTION('center_axis',(-0.707106781186547,8.16340459283203E-17,
-0.707106781186548));
#22916=DIRECTION('ref_axis',(-0.707106781186548,-2.19944674621426E-33,0.707106781186547));
#22917=DIRECTION('',(1.00005772398645E-12,1.,1.00005772398645E-12));
#22918=DIRECTION('center_axis',(0.,-1.,0.));
#22919=DIRECTION('ref_axis',(-0.707106781186548,0.,0.707106781186547));
#22920=DIRECTION('center_axis',(-0.784325130117969,-0.554700196225389,-0.277744095478098));
#22921=DIRECTION('ref_axis',(-0.522883420078948,0.832050294337737,-0.185162730318571));
#22922=DIRECTION('center_axis',(0.,1.,0.));
#22923=DIRECTION('ref_axis',(-0.707106781186548,0.,0.707106781186547));
#22924=DIRECTION('center_axis',(0.784325130117969,-0.554700196225389,-0.277744095478098));
#22925=DIRECTION('ref_axis',(-0.522883420078948,-0.832050294337737,0.185162730318571));
#22926=DIRECTION('',(0.,1.,0.));
#22927=DIRECTION('center_axis',(0.784325130117969,0.554700196225389,-0.277744095478098));
#22928=DIRECTION('ref_axis',(-0.522883420078948,0.832050294337737,0.185162730318571));
#22929=DIRECTION('center_axis',(0.,1.,0.));
#22930=DIRECTION('ref_axis',(-0.707106781186548,0.,0.707106781186547));
#22931=DIRECTION('center_axis',(-0.784325130117969,0.554700196225389,-0.277744095478098));
#22932=DIRECTION('ref_axis',(-0.522883420078948,-0.832050294337737,-0.185162730318571));
#22933=DIRECTION('',(0.,-1.,0.));
#22934=DIRECTION('',(0.,1.,0.));
#22935=DIRECTION('',(0.,-1.,0.));
#22936=DIRECTION('center_axis',(0.942641491092178,0.,0.333806859233771));
#22937=DIRECTION('ref_axis',(0.,-1.,0.));
#22938=DIRECTION('',(0.333806859234345,0.,-0.942641491091975));
#22939=DIRECTION('',(-0.333806859234345,0.,0.942641491091975));
#22940=DIRECTION('',(0.,1.,0.));
#22941=DIRECTION('center_axis',(-0.784325130118311,0.554700196225229,-0.27774409547745));
#22942=DIRECTION('ref_axis',(-0.333806859233771,-9.47580827855939E-17,0.942641491092179));
#22943=DIRECTION('',(0.333806859234345,0.,-0.942641491091975));
#22944=DIRECTION('center_axis',(0.78432513011795,-0.554700196225397,0.277744095478133));
#22945=DIRECTION('ref_axis',(0.522883420078951,0.832050294337732,0.185162730318585));
#22946=DIRECTION('center_axis',(0.,1.,0.));
#22947=DIRECTION('ref_axis',(1.,0.,0.));
#22948=DIRECTION('',(0.333806859234345,0.,0.942641491091975));
#22949=DIRECTION('center_axis',(0.,-1.,0.));
#22950=DIRECTION('ref_axis',(0.707106781186548,0.,-0.707106781186547));
#22951=DIRECTION('center_axis',(0.784325130118311,0.554700196225229,-0.27774409547745));
#22952=DIRECTION('ref_axis',(-1.41728662356081E-16,-0.447721620230319,-0.894172998238226));
#22953=DIRECTION('center_axis',(-0.78432513011795,-0.554700196225398,0.277744095478132));
#22954=DIRECTION('ref_axis',(0.522883420078952,-0.832050294337731,-0.185162730318585));
#22955=DIRECTION('',(-0.333806859234345,0.,-0.942641491091975));
#22956=DIRECTION('center_axis',(-0.942641491092178,0.,0.333806859233771));
#22957=DIRECTION('ref_axis',(0.,1.,0.));
#22958=DIRECTION('',(0.333806859234345,0.,0.942641491091975));
#22959=DIRECTION('',(0.,-1.,0.));
#22960=DIRECTION('center_axis',(0.784325130118311,-0.554700196225229,-0.27774409547745));
#22961=DIRECTION('ref_axis',(-1.41728662356081E-16,0.447721620230319,-0.894172998238226));
#22962=DIRECTION('',(-0.333806859234345,0.,-0.942641491091975));
#22963=DIRECTION('center_axis',(-0.78432513011795,0.554700196225397,0.277744095478133));
#22964=DIRECTION('ref_axis',(0.522883420078951,0.832050294337732,-0.185162730318585));
#22965=DIRECTION('center_axis',(0.,-1.,0.));
#22966=DIRECTION('ref_axis',(0.707106781186548,0.,-0.707106781186547));
#22967=DIRECTION('center_axis',(0.78432513011795,0.554700196225397,0.277744095478133));
#22968=DIRECTION('ref_axis',(0.522883420078951,-0.832050294337732,0.185162730318585));
#22969=DIRECTION('center_axis',(0.,-1.,0.));
#22970=DIRECTION('ref_axis',(0.707106781186548,0.,-0.707106781186547));
#22971=DIRECTION('center_axis',(0.,-1.,0.));
#22972=DIRECTION('ref_axis',(0.,0.,-1.));
#22973=DIRECTION('',(-0.333806859234345,0.,0.942641491091975));
#22974=DIRECTION('center_axis',(-0.784325130118311,-0.554700196225229,-0.27774409547745));
#22975=DIRECTION('ref_axis',(-0.577418677468947,0.816448204670702,1.57337619069903E-16));
#22976=DIRECTION('center_axis',(1.,1.81263994765859E-32,1.11022302462516E-16));
#22977=DIRECTION('ref_axis',(-5.86020957047602E-47,1.,-1.63268091856641E-16));
#22978=DIRECTION('',(1.00011102230146E-12,0.,-1.));
#22979=DIRECTION('',(1.00016326809086E-12,-1.,9.99999999999E-13));
#22980=DIRECTION('',(1.00011102230146E-12,0.,-1.));
#22981=DIRECTION('center_axis',(1.85037170770859E-16,0.,-1.));
#22982=DIRECTION('ref_axis',(-1.,0.,-1.85037170770859E-16));
#22983=DIRECTION('',(1.00011102230146E-12,0.,-1.));
#22984=DIRECTION('center_axis',(6.66685170379299E-12,0.,-1.));
#22985=DIRECTION('ref_axis',(-1.,0.,-6.66685170379299E-12));
#22986=DIRECTION('center_axis',(9.25185853854296E-17,0.,-1.));
#22987=DIRECTION('ref_axis',(1.,0.,9.25185853854296E-17));
#22988=DIRECTION('center_axis',(6.66675918520761E-12,0.,-1.));
#22989=DIRECTION('ref_axis',(1.,0.,6.66675918520761E-12));
#22990=DIRECTION('',(1.00011102230146E-12,0.,-1.));
#22991=DIRECTION('center_axis',(-1.,8.16340459283203E-17,-1.11022302462516E-16));
#22992=DIRECTION('ref_axis',(-1.11022302462516E-16,0.,1.));
#22993=DIRECTION('',(1.00008163404493E-12,1.,9.99999999999E-13));
#22994=DIRECTION('center_axis',(0.,-1.,0.));
#22995=DIRECTION('ref_axis',(-1.51566283225277E-16,0.,1.));
#22996=DIRECTION('center_axis',(-0.75099635150825,-0.554700196225404,0.3582068848149));
#22997=DIRECTION('ref_axis',(-0.500664234338953,0.832050294337727,0.238804589876937));
#22998=DIRECTION('center_axis',(0.,1.,0.));
#22999=DIRECTION('ref_axis',(-6.82745422938049E-13,0.,1.));
#23000=DIRECTION('center_axis',(0.3582068848149,-0.554700196225404,-0.75099635150825));
#23001=DIRECTION('ref_axis',(-0.238804589876937,-0.832050294337727,0.500664234338952));
#23002=DIRECTION('',(0.,1.,0.));
#23003=DIRECTION('center_axis',(0.3582068848149,0.554700196225404,-0.75099635150825));
#23004=DIRECTION('ref_axis',(-0.238804589876937,0.832050294337727,0.500664234338953));
#23005=DIRECTION('center_axis',(0.,1.,0.));
#23006=DIRECTION('ref_axis',(-6.82745422938049E-13,0.,1.));
#23007=DIRECTION('center_axis',(-0.75099635150825,0.554700196225404,0.3582068848149));
#23008=DIRECTION('ref_axis',(-0.500664234338953,-0.832050294337727,0.238804589876937));
#23009=DIRECTION('',(0.,-1.,0.));
#23010=DIRECTION('',(0.,1.,0.));
#23011=DIRECTION('',(0.,-1.,0.));
#23012=DIRECTION('center_axis',(0.902585284349861,0.,-0.430511096808295));
#23013=DIRECTION('ref_axis',(0.,-1.,0.));
#23014=DIRECTION('',(-0.430511096808721,0.,-0.902585284349657));
#23015=DIRECTION('',(0.430511096808721,0.,0.902585284349657));
#23016=DIRECTION('',(0.,1.,0.));
#23017=DIRECTION('center_axis',(-0.750996351508308,0.554700196225229,0.35820688481505));
#23018=DIRECTION('ref_axis',(0.430511096808295,-9.35899339744592E-17,0.902585284349861));
#23019=DIRECTION('',(-0.430511096808721,0.,-0.902585284349657));
#23020=DIRECTION('center_axis',(0.750996351508247,-0.554700196225413,-0.358206884814892));
#23021=DIRECTION('ref_axis',(0.500664234338957,0.832050294337721,-0.238804589876949));
#23022=DIRECTION('center_axis',(0.,1.,0.));
#23023=DIRECTION('ref_axis',(1.,0.,0.));
#23024=DIRECTION('',(0.902585284349657,0.,0.430511096808721));
#23025=DIRECTION('center_axis',(0.,-1.,0.));
#23026=DIRECTION('ref_axis',(7.19584204751227E-13,0.,-1.));
#23027=DIRECTION('center_axis',(0.35820688481505,0.554700196225229,-0.750996351508308));
#23028=DIRECTION('ref_axis',(-0.902585284349861,8.75902672829316E-17,-0.430511096808295));
#23029=DIRECTION('center_axis',(-0.358206884814892,-0.554700196225414,0.750996351508247));
#23030=DIRECTION('ref_axis',(0.23880458987695,-0.83205029433772,-0.500664234338957));
#23031=DIRECTION('',(-0.902585284349657,0.,-0.430511096808721));
#23032=DIRECTION('center_axis',(-0.430511096808295,0.,0.902585284349861));
#23033=DIRECTION('ref_axis',(0.,1.,0.));
#23034=DIRECTION('',(0.902585284349657,0.,0.430511096808721));
#23035=DIRECTION('',(0.,-1.,0.));
#23036=DIRECTION('center_axis',(0.35820688481505,-0.554700196225229,-0.750996351508308));
#23037=DIRECTION('ref_axis',(-4.41754862127715E-17,-0.804372725796521,0.594125001994256));
#23038=DIRECTION('',(-0.902585284349657,0.,-0.430511096808721));
#23039=DIRECTION('center_axis',(-0.358206884814892,0.554700196225413,0.750996351508247));
#23040=DIRECTION('ref_axis',(0.238804589876949,0.832050294337721,-0.500664234338957));
#23041=DIRECTION('center_axis',(0.,-1.,0.));
#23042=DIRECTION('ref_axis',(1.59744320089951E-16,0.,-1.));
#23043=DIRECTION('center_axis',(0.750996351508247,0.554700196225413,-0.358206884814892));
#23044=DIRECTION('ref_axis',(0.500664234338957,-0.832050294337721,-0.238804589876949));
#23045=DIRECTION('center_axis',(0.,-1.,0.));
#23046=DIRECTION('ref_axis',(7.19584204751227E-13,0.,-1.));
#23047=DIRECTION('center_axis',(0.,-1.,0.));
#23048=DIRECTION('ref_axis',(0.,0.,-1.));
#23049=DIRECTION('',(0.430511096808721,0.,0.902585284349657));
#23050=DIRECTION('center_axis',(-0.750996351508308,-0.554700196225229,0.35820688481505));
#23051=DIRECTION('ref_axis',(-0.594125001994256,0.804372725796521,4.34111046316595E-17));
#23052=DIRECTION('center_axis',(0.707106781186548,1.63268091856641E-16,
-0.707106781186547));
#23053=DIRECTION('ref_axis',(7.68102127765282E-32,-1.,-2.30895949806438E-16));
#23054=DIRECTION('',(-0.707106781186547,0.,-0.707106781186548));
#23055=DIRECTION('',(1.0001154479739E-12,-1.,-1.0001154479739E-12));
#23056=DIRECTION('',(-0.707106781186547,0.,-0.707106781186548));
#23057=DIRECTION('center_axis',(-0.707106781186547,0.,-0.707106781186548));
#23058=DIRECTION('ref_axis',(-0.707106781186548,0.,0.707106781186547));
#23059=DIRECTION('',(-0.707106781186547,0.,-0.707106781186548));
#23060=DIRECTION('center_axis',(-0.707106781186547,0.,-0.707106781186548));
#23061=DIRECTION('ref_axis',(-0.707106781186548,0.,0.707106781186547));
#23062=DIRECTION('center_axis',(-0.707106781186547,0.,-0.707106781186548));
#23063=DIRECTION('ref_axis',(0.707106781186548,0.,-0.707106781186547));
#23064=DIRECTION('center_axis',(-0.707106781186547,0.,-0.707106781186548));
#23065=DIRECTION('ref_axis',(0.707106781186548,0.,-0.707106781186547));
#23066=DIRECTION('',(-0.707106781186547,0.,-0.707106781186548));
#23067=DIRECTION('center_axis',(-0.707106781186548,8.16340459283203E-17,
0.707106781186547));
#23068=DIRECTION('ref_axis',(1.15447974903219E-16,1.,1.84458295290239E-31));
#23069=DIRECTION('',(1.00005772398645E-12,1.,-1.00005772398645E-12));
#23070=DIRECTION('center_axis',(0.,-1.,0.));
#23071=DIRECTION('ref_axis',(0.707106781186547,0.,0.707106781186548));
#23072=DIRECTION('center_axis',(-0.277744095478098,-0.554700196225389,0.784325130117969));
#23073=DIRECTION('ref_axis',(-0.185162730318571,0.832050294337737,0.522883420078948));
#23074=DIRECTION('center_axis',(0.,1.,0.));
#23075=DIRECTION('ref_axis',(0.707106781186547,0.,0.707106781186548));
#23076=DIRECTION('center_axis',(-0.277744095478098,-0.554700196225389,-0.784325130117969));
#23077=DIRECTION('ref_axis',(0.185162730318571,-0.832050294337737,0.522883420078948));
#23078=DIRECTION('',(0.,1.,0.));
#23079=DIRECTION('center_axis',(-0.277744095478098,0.554700196225389,-0.784325130117969));
#23080=DIRECTION('ref_axis',(0.185162730318571,0.832050294337737,0.522883420078948));
#23081=DIRECTION('center_axis',(0.,1.,0.));
#23082=DIRECTION('ref_axis',(0.707106781186547,0.,0.707106781186548));
#23083=DIRECTION('center_axis',(-0.277744095478098,0.554700196225389,0.784325130117969));
#23084=DIRECTION('ref_axis',(-0.185162730318571,-0.832050294337737,0.522883420078948));
#23085=DIRECTION('',(0.,-1.,0.));
#23086=DIRECTION('',(0.,1.,0.));
#23087=DIRECTION('',(0.,-1.,0.));
#23088=DIRECTION('center_axis',(0.333806859233771,0.,-0.942641491092178));
#23089=DIRECTION('ref_axis',(0.,-1.,0.));
#23090=DIRECTION('',(-0.942641491091975,0.,-0.333806859234345));
#23091=DIRECTION('',(0.942641491091975,0.,0.333806859234345));
#23092=DIRECTION('',(0.,1.,0.));
#23093=DIRECTION('center_axis',(-0.27774409547745,0.554700196225229,0.784325130118311));
#23094=DIRECTION('ref_axis',(0.894172998238226,0.447721620230319,1.29766088156978E-16));
#23095=DIRECTION('',(-0.942641491091975,0.,-0.333806859234345));
#23096=DIRECTION('center_axis',(0.277744095478133,-0.554700196225397,-0.78432513011795));
#23097=DIRECTION('ref_axis',(0.185162730318585,0.832050294337732,-0.522883420078951));
#23098=DIRECTION('center_axis',(0.,1.,0.));
#23099=DIRECTION('ref_axis',(1.,0.,0.));
#23100=DIRECTION('',(0.942641491091975,0.,-0.333806859234345));
#23101=DIRECTION('center_axis',(0.,-1.,0.));
#23102=DIRECTION('ref_axis',(-0.707106781186547,0.,-0.707106781186548));
#23103=DIRECTION('center_axis',(-0.27774409547745,0.554700196225229,-0.784325130118311));
#23104=DIRECTION('ref_axis',(-0.942641491092179,8.22449654774124E-17,0.333806859233771));
#23105=DIRECTION('center_axis',(0.277744095478132,-0.554700196225398,0.78432513011795));
#23106=DIRECTION('ref_axis',(-0.185162730318585,-0.832050294337731,-0.522883420078952));
#23107=DIRECTION('',(-0.942641491091975,0.,0.333806859234345));
#23108=DIRECTION('center_axis',(0.333806859233771,0.,0.942641491092178));
#23109=DIRECTION('ref_axis',(0.,-1.,0.));
#23110=DIRECTION('',(0.942641491091975,0.,-0.333806859234345));
#23111=DIRECTION('',(0.,-1.,0.));
#23112=DIRECTION('center_axis',(-0.27774409547745,-0.554700196225229,-0.784325130118311));
#23113=DIRECTION('ref_axis',(-1.53589745588664E-16,-0.816448204670702,0.577418677468947));
#23114=DIRECTION('',(-0.942641491091975,0.,0.333806859234345));
#23115=DIRECTION('center_axis',(0.277744095478133,0.554700196225397,0.78432513011795));
#23116=DIRECTION('ref_axis',(-0.185162730318585,0.832050294337732,-0.522883420078951));
#23117=DIRECTION('center_axis',(0.,-1.,0.));
#23118=DIRECTION('ref_axis',(-0.707106781186547,0.,-0.707106781186548));
#23119=DIRECTION('center_axis',(0.277744095478133,0.554700196225397,-0.78432513011795));
#23120=DIRECTION('ref_axis',(0.185162730318585,-0.832050294337732,-0.522883420078951));
#23121=DIRECTION('center_axis',(0.,-1.,0.));
#23122=DIRECTION('ref_axis',(-0.707106781186547,0.,-0.707106781186548));
#23123=DIRECTION('center_axis',(0.,-1.,0.));
#23124=DIRECTION('ref_axis',(0.,0.,-1.));
#23125=DIRECTION('',(0.942641491091975,0.,0.333806859234345));
#23126=DIRECTION('center_axis',(-0.27774409547745,-0.554700196225229,0.784325130118311));
#23127=DIRECTION('ref_axis',(-0.894172998238226,0.447721620230319,-1.29766088156978E-16));
#23128=DIRECTION('center_axis',(1.11022302462516E-16,1.63268091856641E-16,
-1.));
#23129=DIRECTION('ref_axis',(-1.,-1.12696337893758E-48,-1.11022302462516E-16));
#23130=DIRECTION('',(-1.,0.,-1.00011102230146E-12));
#23131=DIRECTION('',(9.99999999999E-13,-1.,-1.00016326809086E-12));
#23132=DIRECTION('',(-1.,0.,-1.00011102230146E-12));
#23133=DIRECTION('center_axis',(-1.,0.,-1.85037170770859E-16));
#23134=DIRECTION('ref_axis',(-1.85037170770859E-16,0.,1.));
#23135=DIRECTION('',(-1.,0.,-1.00011102230146E-12));
#23136=DIRECTION('center_axis',(-1.,0.,-6.66685170379299E-12));
#23137=DIRECTION('ref_axis',(-6.66685170379299E-12,0.,1.));
#23138=DIRECTION('center_axis',(-1.,0.,-2.77555756156289E-16));
#23139=DIRECTION('ref_axis',(2.77555756156289E-16,0.,-1.));
#23140=DIRECTION('center_axis',(-1.,0.,-6.66694422237838E-12));
#23141=DIRECTION('ref_axis',(6.66694422237838E-12,0.,-1.));
#23142=DIRECTION('center_axis',(-1.,0.,-6.66694422237838E-12));
#23143=DIRECTION('ref_axis',(6.66694422237838E-12,0.,-1.));
#23144=DIRECTION('center_axis',(-1.,0.,-6.66694422237838E-12));
#23145=DIRECTION('ref_axis',(6.66694422237838E-12,0.,-1.));
#23146=DIRECTION('',(-1.,0.,-1.00011102230146E-12));
#23147=DIRECTION('center_axis',(-9.0631997382929E-33,8.16340459283203E-17,
1.));
#23148=DIRECTION('ref_axis',(1.,1.11022302462516E-16,5.6348168946886E-49));
#23149=DIRECTION('',(9.99999999999E-13,1.,-1.00008163404493E-12));
#23150=DIRECTION('center_axis',(0.,1.,0.));
#23151=DIRECTION('ref_axis',(1.,0.,0.));
#23152=DIRECTION('',(1.00027992850901E-12,0.,-1.));
#23153=DIRECTION('',(-0.707106781186547,0.,-0.707106781186548));
#23154=DIRECTION('',(-1.,0.,-1.00027992850901E-12));
#23155=DIRECTION('',(-0.707106781186548,0.,0.707106781186547));
#23156=DIRECTION('',(1.00027992850901E-12,0.,1.));
#23157=DIRECTION('',(0.707106781186547,0.,0.707106781186548));
#23158=DIRECTION('',(1.,0.,1.00027992850901E-12));
#23159=DIRECTION('',(0.707106781186548,0.,-0.707106781186547));
#23160=DIRECTION('',(-1.00029133863849E-12,0.,1.));
#23161=DIRECTION('',(-0.707106781186548,0.,0.707106781186548));
#23162=DIRECTION('',(-1.,0.,0.));
#23163=DIRECTION('',(-0.707106781186548,0.,-0.707106781186547));
#23164=DIRECTION('',(1.00014566931874E-12,0.,-1.));
#23165=DIRECTION('',(0.707106781186547,0.,-0.707106781186548));
#23166=DIRECTION('',(1.,0.,0.));
#23167=DIRECTION('',(0.707106781186548,0.,0.707106781186548));
#23168=DIRECTION('center_axis',(-0.707106781186548,0.,0.707106781186547));
#23169=DIRECTION('ref_axis',(0.,1.,0.));
#23170=DIRECTION('',(0.,1.,0.));
#23171=DIRECTION('',(0.,-1.,0.));
#23172=DIRECTION('',(-0.707106781186547,0.,-0.707106781186548));
#23173=DIRECTION('center_axis',(-2.19351898461705E-47,7.8359970714266E-32,
1.));
#23174=DIRECTION('ref_axis',(1.,2.79928510006155E-16,7.56996450688685E-62));
#23175=DIRECTION('',(0.,1.,0.));
#23176=DIRECTION('',(-1.,0.,-1.00027992850901E-12));
#23177=DIRECTION('center_axis',(0.707106781186547,0.,0.707106781186548));
#23178=DIRECTION('ref_axis',(0.,-1.,0.));
#23179=DIRECTION('',(0.,1.,0.));
#23180=DIRECTION('',(0.,1.,0.));
#23181=DIRECTION('',(-0.707106781186548,0.,0.707106781186547));
#23182=DIRECTION('center_axis',(0.707106781186548,0.,-0.707106781186547));
#23183=DIRECTION('ref_axis',(0.,-1.,0.));
#23184=DIRECTION('',(0.,1.,0.));
#23185=DIRECTION('',(0.,1.,0.));
#23186=DIRECTION('',(0.,1.,0.));
#23187=DIRECTION('',(0.707106781186547,0.,0.707106781186548));
#23188=DIRECTION('center_axis',(2.79928510006155E-16,0.,-1.));
#23189=DIRECTION('ref_axis',(0.,-1.,0.));
#23190=DIRECTION('',(0.,1.,0.));
#23191=DIRECTION('',(1.,0.,1.00027992850901E-12));
#23192=DIRECTION('center_axis',(-0.707106781186547,0.,-0.707106781186548));
#23193=DIRECTION('ref_axis',(-0.707106781186548,0.,0.707106781186547));
#23194=DIRECTION('',(0.,1.,0.));
#23195=DIRECTION('',(0.707106781186548,0.,-0.707106781186547));
#23196=DIRECTION('center_axis',(-1.,0.,2.79928510006155E-16));
#23197=DIRECTION('ref_axis',(0.,1.,0.));
#23198=DIRECTION('',(-1.00027992850901E-12,0.,-1.));
#23199=DIRECTION('center_axis',(0.,-1.,0.));
#23200=DIRECTION('ref_axis',(0.,0.,-1.));
#23201=DIRECTION('',(1.,0.,1.00027755575516E-12));
#23202=DIRECTION('',(1.00027992850901E-12,1.00002114947192E-12,-1.));
#23203=DIRECTION('',(1.,0.,1.00027755575516E-12));
#23204=DIRECTION('',(-1.,0.,-1.00027992850901E-12));
#23205=DIRECTION('',(1.00029133863849E-12,0.,-1.));
#23206=DIRECTION('',(-0.707106781186548,0.,-0.707106781186548));
#23207=DIRECTION('',(-1.,0.,0.));
#23208=DIRECTION('',(-0.707106781186547,0.,0.707106781186548));
#23209=DIRECTION('',(-1.00014566931874E-12,0.,1.));
#23210=DIRECTION('',(0.707106781186548,0.,0.707106781186547));
#23211=DIRECTION('',(1.,0.,0.));
#23212=DIRECTION('',(0.707106781186548,0.,-0.707106781186548));
#23213=DIRECTION('',(1.00029133863849E-12,0.,-1.));
#23214=DIRECTION('',(1.,0.,1.00027992850901E-12));
#23215=DIRECTION('',(1.00027992850901E-12,0.,-1.));
#23216=DIRECTION('center_axis',(-0.707106781186548,0.,-0.707106781186548));
#23217=DIRECTION('ref_axis',(-0.707106781186548,0.,0.707106781186548));
#23218=DIRECTION('',(0.,1.,0.));
#23219=DIRECTION('',(0.,1.,0.));
#23220=DIRECTION('center_axis',(0.,0.,-1.));
#23221=DIRECTION('ref_axis',(0.,-1.,0.));
#23222=DIRECTION('',(0.,-1.,0.));
#23223=DIRECTION('center_axis',(0.707106781186547,0.,-0.707106781186548));
#23224=DIRECTION('ref_axis',(0.,-1.,0.));
#23225=DIRECTION('',(0.,1.,0.));
#23226=DIRECTION('center_axis',(1.,2.12195507149859E-32,3.0910375179476E-48));
#23227=DIRECTION('ref_axis',(6.6848796930149E-63,-1.45669319745051E-16,
1.));
#23228=DIRECTION('',(0.,1.,0.));
#23229=DIRECTION('center_axis',(0.707106781186548,0.,0.707106781186547));
#23230=DIRECTION('ref_axis',(0.,-1.,0.));
#23231=DIRECTION('',(0.,1.,0.));
#23232=DIRECTION('center_axis',(0.,0.,1.));
#23233=DIRECTION('ref_axis',(1.,0.,0.));
#23234=DIRECTION('',(0.,1.,0.));
#23235=DIRECTION('center_axis',(-0.707106781186548,0.,0.707106781186548));
#23236=DIRECTION('ref_axis',(0.,1.,0.));
#23237=DIRECTION('',(0.,1.,0.));
#23238=DIRECTION('center_axis',(0.,1.,0.));
#23239=DIRECTION('ref_axis',(1.,0.,0.));
#23240=DIRECTION('',(-1.00029133863849E-12,0.,1.));
#23241=DIRECTION('',(-1.,0.,0.));
#23242=DIRECTION('',(1.00027992850901E-12,0.,-1.));
#23243=DIRECTION('',(-1.,0.,0.));
#23244=DIRECTION('',(-1.00029133863849E-12,0.,1.));
#23245=DIRECTION('',(-1.00029133863849E-12,0.,1.));
#23246=DIRECTION('center_axis',(0.,1.5419764230905E-16,-1.));
#23247=DIRECTION('ref_axis',(-1.,0.,0.));
#23248=DIRECTION('',(-1.,0.,0.));
#23249=DIRECTION('',(9.99999999999E-13,-1.,-1.00024671622669E-12));
#23250=DIRECTION('',(1.,0.,1.00027755575516E-12));
#23251=DIRECTION('',(0.,1.,0.));
#23252=DIRECTION('',(0.,1.,0.));
#23253=DIRECTION('center_axis',(0.,0.,1.));
#23254=DIRECTION('ref_axis',(1.,0.,0.));
#23255=DIRECTION('',(1.,0.,1.00027755575516E-12));
#23256=DIRECTION('',(0.,1.,0.));
#23257=DIRECTION('',(-1.,0.,0.));
#23258=DIRECTION('',(0.,1.,0.));
#23259=DIRECTION('',(0.,-1.,0.));
#23260=DIRECTION('center_axis',(-1.,0.,-2.91338639490101E-16));
#23261=DIRECTION('ref_axis',(-2.91338639490101E-16,0.,1.));
#23262=DIRECTION('center_axis',(1.,7.70371977754894E-32,2.13821176807375E-47));
#23263=DIRECTION('ref_axis',(4.61864415153757E-62,-2.77555756156289E-16,
1.));
#23264=DIRECTION('',(-1.00027992850901E-12,0.,1.));
#23265=DIRECTION('',(-1.00027992850901E-12,-1.00015458001819E-12,1.));
#23266=DIRECTION('',(-1.00027992850901E-12,0.,1.));
#23267=DIRECTION('',(9.99999999999001E-13,-1.,-3.55964561715128E-12));
#23268=DIRECTION('',(-9.99999999999E-13,1.,1.00010573552515E-12));
#23269=DIRECTION('center_axis',(0.,1.,0.));
#23270=DIRECTION('ref_axis',(1.,0.,0.));
#23271=DIRECTION('',(1.00027992850901E-12,0.,-1.));
#23272=DIRECTION('',(1.,0.,1.00027755575516E-12));
#23273=DIRECTION('center_axis',(0.,1.,0.));
#23274=DIRECTION('ref_axis',(1.,0.,0.));
#23275=DIRECTION('',(1.00027992850901E-12,0.,-1.));
#23276=DIRECTION('',(1.,0.,1.00027755575516E-12));
#23277=DIRECTION('center_axis',(7.10444374761543E-28,-2.55964561715484E-12,
1.));
#23278=DIRECTION('ref_axis',(1.,2.77555756156289E-16,-3.7860081723633E-43));
#23279=DIRECTION('center_axis',(2.77555756156289E-16,1.05735526154777E-16,
-1.));
#23280=DIRECTION('ref_axis',(0.,-1.,-1.05735526154777E-16));
#23281=DIRECTION('center_axis',(-1.,0.,-2.91338639490101E-16));
#23282=DIRECTION('ref_axis',(-2.91338639490101E-16,0.,1.));
#23283=DIRECTION('center_axis',(1.,7.8359970714266E-32,2.19351898461705E-47));
#23284=DIRECTION('ref_axis',(-7.77876909732643E-62,-2.79928510006155E-16,
1.));
#23285=DIRECTION('center_axis',(0.,-1.,-1.2559626558816E-16));
#23286=DIRECTION('ref_axis',(0.,1.2559626558816E-16,-1.));
#23287=DIRECTION('',(-1.00027992850901E-12,-1.00012559626459E-12,1.));
#23288=DIRECTION('center_axis',(1.,7.8359970714266E-32,2.19351898461705E-47));
#23289=DIRECTION('ref_axis',(-7.77876909732643E-62,-2.79928510006155E-16,
1.));
#28721=CARTESIAN_POINT('',(0.,0.,0.));
#28722=CARTESIAN_POINT('Origin',(-4.56515315114362E-17,-0.00365,-6.77116287837691E-17));
#28723=CARTESIAN_POINT('',(0.0116511274118543,-0.02925,-0.00888108833605083));
#28724=CARTESIAN_POINT('',(0.0132228744157255,-0.02475,-0.0063069875682416));
#28725=CARTESIAN_POINT('Origin',(-4.56515315114362E-17,-0.02475000000001,
-6.77116287837691E-17));
#28726=CARTESIAN_POINT('',(0.00888108833605071,-0.02925,-0.0116511274118544));
#28727=CARTESIAN_POINT('Origin',(-4.56515315114362E-17,-0.02925000000001,
-6.77116287837691E-17));
#28728=CARTESIAN_POINT('',(0.00630698756824148,-0.02475,-0.0132228744157256));
#28729=CARTESIAN_POINT('Origin',(-4.56515315114362E-17,-0.02475000000001,
-6.77116287837691E-17));
#28730=CARTESIAN_POINT('',(0.00630698756824148,-0.00815,-0.0132228744157256));
#28731=CARTESIAN_POINT('',(0.00630698756825148,-0.00364999999999,-0.0132228744157356));
#28732=CARTESIAN_POINT('',(0.00888108833605071,-0.00365,-0.0116511274118544));
#28733=CARTESIAN_POINT('Origin',(-4.56515315114362E-17,-0.00814999999999,
-6.77116287837691E-17));
#28734=CARTESIAN_POINT('',(0.0116511274118543,-0.00365,-0.00888108833605083));
#28735=CARTESIAN_POINT('Origin',(-4.56515315114362E-17,-0.00364999999999,
-6.77116287837691E-17));
#28736=CARTESIAN_POINT('',(0.0132228744157255,-0.00815,-0.0063069875682416));
#28737=CARTESIAN_POINT('Origin',(-4.56515315114362E-17,-0.00814999999999,
-6.77116287837691E-17));
#28738=CARTESIAN_POINT('',(0.0132228744157355,-0.00364999999999,-0.0063069875682516));
#28739=CARTESIAN_POINT('',(0.0113653314426162,-0.02325,-0.0092440110990566));
#28740=CARTESIAN_POINT('',(0.0113653314426162,-0.00965,-0.0092440110990566));
#28741=CARTESIAN_POINT('',(0.0113653314426262,-0.00364999999999,-0.0092440110990666));
#28742=CARTESIAN_POINT('',(0.00924401109905649,-0.00965,-0.0113653314426163));
#28743=CARTESIAN_POINT('Ctrl Pts',(0.0113653314426161,-0.00965,-0.00924401109905659));
#28744=CARTESIAN_POINT('Ctrl Pts',(0.0113653314426161,-0.00946151448459537,
-0.00924401109905659));
#28745=CARTESIAN_POINT('Ctrl Pts',(0.0113415286147626,-0.00926055630226628,
-0.00927351838063712));
#28746=CARTESIAN_POINT('Ctrl Pts',(0.0112435430943065,-0.00889102670991339,
-0.00939207927644872));
#28747=CARTESIAN_POINT('Ctrl Pts',(0.011169215384428,-0.00872244398548004,
-0.00948097768002299));
#28748=CARTESIAN_POINT('Ctrl Pts',(0.010994642278187,-0.00845623616911263,
-0.00968287927809851));
#28749=CARTESIAN_POINT('Ctrl Pts',(0.0108827047851676,-0.00834081748849188,
-0.00980935406895069));
#28750=CARTESIAN_POINT('Ctrl Pts',(0.010631656844134,-0.00818769575944871,
-0.0100809009239758));
#28751=CARTESIAN_POINT('Ctrl Pts',(0.0104923932316728,-0.00815,-0.010225835457093));
#28752=CARTESIAN_POINT('Ctrl Pts',(0.0102258354570929,-0.00815,-0.0104923932316729));
#28753=CARTESIAN_POINT('Ctrl Pts',(0.0100809009239757,-0.00818769575944871,
-0.0106316568441341));
#28754=CARTESIAN_POINT('Ctrl Pts',(0.00980935406895059,-0.00834081748849188,
-0.0108827047851677));
#28755=CARTESIAN_POINT('Ctrl Pts',(0.00968287927809842,-0.00845623616911263,
-0.0109946422781871));
#28756=CARTESIAN_POINT('Ctrl Pts',(0.0094809776800229,-0.00872244398548004,
-0.0111692153844281));
#28757=CARTESIAN_POINT('Ctrl Pts',(0.00939207927644862,-0.00889102670991339,
-0.0112435430943066));
#28758=CARTESIAN_POINT('Ctrl Pts',(0.00927351838063703,-0.00926055630226629,
-0.0113415286147627));
#28759=CARTESIAN_POINT('Ctrl Pts',(0.00924401109905649,-0.00946151448459537,
-0.0113653314426162));
#28760=CARTESIAN_POINT('Ctrl Pts',(0.00924401109905649,-0.00965,-0.0113653314426162));
#28761=CARTESIAN_POINT('',(0.00924401109905649,-0.02325,-0.0113653314426163));
#28762=CARTESIAN_POINT('',(0.00924401109906649,-0.00364999999999,-0.0113653314426263));
#28763=CARTESIAN_POINT('Ctrl Pts',(0.00924401109905649,-0.02325,-0.0113653314426162));
#28764=CARTESIAN_POINT('Ctrl Pts',(0.00924401109905649,-0.0234384855154046,
-0.0113653314426162));
#28765=CARTESIAN_POINT('Ctrl Pts',(0.00927351838063703,-0.0236394436977337,
-0.0113415286147627));
#28766=CARTESIAN_POINT('Ctrl Pts',(0.00939207927644862,-0.0240089732900866,
-0.0112435430943066));
#28767=CARTESIAN_POINT('Ctrl Pts',(0.0094809776800229,-0.02417755601452,
-0.0111692153844281));
#28768=CARTESIAN_POINT('Ctrl Pts',(0.00968287927809842,-0.0244437638308874,
-0.0109946422781871));
#28769=CARTESIAN_POINT('Ctrl Pts',(0.00980935406895059,-0.0245591825115081,
-0.0108827047851677));
#28770=CARTESIAN_POINT('Ctrl Pts',(0.0100809009239757,-0.0247123042405513,
-0.0106316568441341));
#28771=CARTESIAN_POINT('Ctrl Pts',(0.0102258354570929,-0.02475,-0.0104923932316729));
#28772=CARTESIAN_POINT('Ctrl Pts',(0.0104923932316728,-0.02475,-0.010225835457093));
#28773=CARTESIAN_POINT('Ctrl Pts',(0.010631656844134,-0.0247123042405513,
-0.0100809009239758));
#28774=CARTESIAN_POINT('Ctrl Pts',(0.0108827047851676,-0.0245591825115081,
-0.00980935406895069));
#28775=CARTESIAN_POINT('Ctrl Pts',(0.010994642278187,-0.0244437638308874,
-0.00968287927809851));
#28776=CARTESIAN_POINT('Ctrl Pts',(0.011169215384428,-0.02417755601452,
-0.00948097768002299));
#28777=CARTESIAN_POINT('Ctrl Pts',(0.0112435430943065,-0.0240089732900866,
-0.00939207927644872));
#28778=CARTESIAN_POINT('Ctrl Pts',(0.0113415286147626,-0.0236394436977337,
-0.00927351838063713));
#28779=CARTESIAN_POINT('Ctrl Pts',(0.0113653314426161,-0.0234384855154046,
-0.00924401109905659));
#28780=CARTESIAN_POINT('Ctrl Pts',(0.0113653314426161,-0.02325,-0.00924401109905659));
#28781=CARTESIAN_POINT('Origin',(0.0125459354524631,-0.00365,-0.00598410424563538));
#28782=CARTESIAN_POINT('',(0.0125459354524631,-0.02475,-0.00598410424563538));
#28783=CARTESIAN_POINT('',(0.00627296772624148,-0.02475000000001,-0.00299205212282772));
#28784=CARTESIAN_POINT('',(0.0125459354524631,-0.00815,-0.00598410424563538));
#28785=CARTESIAN_POINT('',(0.00627296772624148,-0.00814999999999,-0.00299205212282772));
#28786=CARTESIAN_POINT('',(0.0125459354524731,-0.00364999999999,-0.00598410424564538));
#28787=CARTESIAN_POINT('Origin',(0.00562720108101904,-0.0059,-0.00434593004934251));
#28788=CARTESIAN_POINT('',(0.0109587138343332,-0.00365,-0.00855082400106528));
#28789=CARTESIAN_POINT('',(0.00498143443581659,-0.00364999999999,-0.0056998079758773));
#28790=CARTESIAN_POINT('Origin',(-4.56515315114362E-17,-0.00814999999999,
-6.77116287837691E-17));
#28791=CARTESIAN_POINT('Origin',(-4.56515315114362E-17,-0.00365,-6.77116287837691E-17));
#28792=CARTESIAN_POINT('',(0.00855082400106516,-0.00365,-0.0109587138343334));
#28793=CARTESIAN_POINT('',(0.00586124963718029,-0.00364999999999,-0.00531990391744792));
#28794=CARTESIAN_POINT('Origin',(-4.56515315114362E-17,-0.00364999999999,
-6.77116287837691E-17));
#28795=CARTESIAN_POINT('Origin',(0.0045073717106455,-0.0059,-0.00596567056265036));
#28796=CARTESIAN_POINT('',(0.00598410424563526,-0.00815,-0.0125459354524632));
#28797=CARTESIAN_POINT('Origin',(-4.56515315114362E-17,-0.00814999999999,
-6.77116287837691E-17));
#28798=CARTESIAN_POINT('',(0.00315349378413072,-0.00814999999999,-0.0066114372078728));
#28799=CARTESIAN_POINT('Origin',(0.00630698756824148,-0.00365,-0.0132228744157256));
#28800=CARTESIAN_POINT('',(0.00598410424563526,-0.02475,-0.0125459354524632));
#28801=CARTESIAN_POINT('',(0.00315349378413072,-0.02475000000001,-0.0066114372078728));
#28802=CARTESIAN_POINT('',(0.00598410424564526,-0.00364999999999,-0.0125459354524732));
#28803=CARTESIAN_POINT('Origin',(0.0045073717106455,-0.027,-0.00596567056265036));
#28804=CARTESIAN_POINT('',(0.00855082400106516,-0.02925,-0.0109587138343334));
#28805=CARTESIAN_POINT('',(0.00586124963718029,-0.02925000000001,-0.00531990391744792));
#28806=CARTESIAN_POINT('Origin',(-4.56515315114362E-17,-0.02475000000001,
-6.77116287837691E-17));
#28807=CARTESIAN_POINT('Origin',(-4.56515315114362E-17,-0.00365,-6.77116287837691E-17));
#28808=CARTESIAN_POINT('',(0.0109587138343332,-0.02925,-0.00855082400106528));
#28809=CARTESIAN_POINT('Origin',(-4.56515315114362E-17,-0.02475000000001,
-6.77116287837691E-17));
#28810=CARTESIAN_POINT('Origin',(-4.56515315114362E-17,-0.02925000000001,
-6.77116287837691E-17));
#28811=CARTESIAN_POINT('Origin',(-4.56515315114362E-17,-0.02925,-6.77116287837691E-17));
#28812=CARTESIAN_POINT('',(0.00498143443581659,-0.02925000000001,-0.0056998079758773));
#28813=CARTESIAN_POINT('Origin',(0.00562720108101904,-0.027,-0.00434593004934251));
#28814=CARTESIAN_POINT('Origin',(0.0119501046020527,-0.00965,-0.0140714249456124));
#28815=CARTESIAN_POINT('',(0.0119501046020527,-0.00965,-0.0140714249456124));
#28816=CARTESIAN_POINT('',(0.0119501046020627,-0.00964999999999,-0.0140714249456224));
#28817=CARTESIAN_POINT('',(0.0119501046020527,-0.02325,-0.0140714249456124));
#28818=CARTESIAN_POINT('',(0.0119501046020627,-0.00964999999999,-0.0140714249456224));
#28819=CARTESIAN_POINT('',(0.0119501046020627,-0.02325000000001,-0.0140714249456224));
#28820=CARTESIAN_POINT('Origin',(0.0130107647738325,-0.00965,-0.0130107647738326));
#28821=CARTESIAN_POINT('',(0.0140714249456123,-0.00965,-0.0119501046020528));
#28822=CARTESIAN_POINT('',(0.0140714249456223,-0.00964999999999,-0.0119501046020628));
#28823=CARTESIAN_POINT('Origin',(0.0130107647738425,-0.00964999999999,-0.0130107647738426));
#28824=CARTESIAN_POINT('Origin',(0.0130107647738325,-0.02325,-0.0130107647738326));
#28825=CARTESIAN_POINT('',(0.0140714249456123,-0.02325,-0.0119501046020528));
#28826=CARTESIAN_POINT('Origin',(0.0130107647738425,-0.02325000000001,-0.0130107647738426));
#28827=CARTESIAN_POINT('',(0.0140714249456223,-0.02325000000001,-0.0119501046020628));
#28828=CARTESIAN_POINT('Origin',(0.0140714249456123,-0.02325,-0.0119501046020528));
#28829=CARTESIAN_POINT('',(0.0140714249456223,-0.02325000000001,-0.0119501046020628));
#28830=CARTESIAN_POINT('Origin',(-4.56515315114362E-17,-0.00365,-6.77116287837691E-17));
#28831=CARTESIAN_POINT('',(0.00195871341465237,-0.02925,-0.014518468988129));
#28832=CARTESIAN_POINT('',(0.00489027048777469,-0.02475,-0.0138096978445005));
#28833=CARTESIAN_POINT('Origin',(-4.56515315114362E-17,-0.02475000000001,
-6.77116287837691E-17));
#28834=CARTESIAN_POINT('',(-0.00195871341465248,-0.02925,-0.014518468988129));
#28835=CARTESIAN_POINT('Origin',(-4.56515315114362E-17,-0.02925000000001,
-6.77116287837691E-17));
#28836=CARTESIAN_POINT('',(-0.0048902704877748,-0.02475,-0.0138096978445005));
#28837=CARTESIAN_POINT('Origin',(-4.56515315114362E-17,-0.02475000000001,
-6.77116287837691E-17));
#28838=CARTESIAN_POINT('',(-0.0048902704877748,-0.00815,-0.0138096978445005));
#28839=CARTESIAN_POINT('',(-0.0048902704877848,-0.00364999999999,-0.0138096978445105));
#28840=CARTESIAN_POINT('',(-0.00195871341465248,-0.00365,-0.014518468988129));
#28841=CARTESIAN_POINT('Origin',(-4.56515315114362E-17,-0.00814999999999,
-6.77116287837691E-17));
#28842=CARTESIAN_POINT('',(0.00195871341465237,-0.00365,-0.014518468988129));
#28843=CARTESIAN_POINT('Origin',(-4.56515315114362E-17,-0.00364999999999,
-6.77116287837691E-17));
#28844=CARTESIAN_POINT('',(0.00489027048777469,-0.00815,-0.0138096978445005));
#28845=CARTESIAN_POINT('Origin',(-4.56515315114362E-17,-0.00814999999999,
-6.77116287837691E-17));
#28846=CARTESIAN_POINT('',(0.00489027048778469,-0.00364999999999,-0.0138096978445105));
#28847=CARTESIAN_POINT('',(0.00149999999999995,-0.02325,-0.0145730058670133));
#28848=CARTESIAN_POINT('',(0.00149999999999995,-0.00965,-0.0145730058670133));
#28849=CARTESIAN_POINT('',(0.00150000000000995,-0.00364999999999,-0.0145730058670233));
#28850=CARTESIAN_POINT('',(-0.00150000000000005,-0.00965,-0.0145730058670133));
#28851=CARTESIAN_POINT('Ctrl Pts',(0.00149999999999995,-0.00965,-0.0145730058670132));
#28852=CARTESIAN_POINT('Ctrl Pts',(0.00149999999999995,-0.00946151448459537,
-0.0145730058670132));
#28853=CARTESIAN_POINT('Ctrl Pts',(0.00146230406011329,-0.00926055630226629,
-0.0145770395249265));
#28854=CARTESIAN_POINT('Ctrl Pts',(0.00130918262072881,-0.00889102670991339,
-0.0145915885123659));
#28855=CARTESIAN_POINT('Ctrl Pts',(0.00119376432903963,-0.00872244398548004,
-0.0146018915486848));
#28856=CARTESIAN_POINT('Ctrl Pts',(0.000927556512672221,-0.00845623616911263,
-0.0146212157105806));
#28857=CARTESIAN_POINT('Ctrl Pts',(0.000758973570028426,-0.00834081748849188,
-0.0146314951324582));
#28858=CARTESIAN_POINT('Ctrl Pts',(0.000389443245922543,-0.00818769575944871,
-0.0146459900535486));
#28859=CARTESIAN_POINT('Ctrl Pts',(0.000188484809983391,-0.00815,-0.0146500000000001));
#28860=CARTESIAN_POINT('Ctrl Pts',(-0.000188484809983482,-0.00815,-0.0146500000000001));
#28861=CARTESIAN_POINT('Ctrl Pts',(-0.000389443245922634,-0.00818769575944871,
-0.0146459900535486));
#28862=CARTESIAN_POINT('Ctrl Pts',(-0.000758973570028517,-0.00834081748849188,
-0.0146314951324582));
#28863=CARTESIAN_POINT('Ctrl Pts',(-0.000927556512672312,-0.00845623616911263,
-0.0146212157105806));
#28864=CARTESIAN_POINT('Ctrl Pts',(-0.00119376432903972,-0.00872244398548004,
-0.0146018915486848));
#28865=CARTESIAN_POINT('Ctrl Pts',(-0.0013091826207289,-0.00889102670991339,
-0.0145915885123659));
#28866=CARTESIAN_POINT('Ctrl Pts',(-0.00146230406011339,-0.00926055630226629,
-0.0145770395249265));
#28867=CARTESIAN_POINT('Ctrl Pts',(-0.00150000000000005,-0.00946151448459537,
-0.0145730058670132));
#28868=CARTESIAN_POINT('Ctrl Pts',(-0.00150000000000005,-0.00965,-0.0145730058670132));
#28869=CARTESIAN_POINT('',(-0.00150000000000005,-0.02325,-0.0145730058670133));
#28870=CARTESIAN_POINT('',(-0.00150000000001003,-0.00364999999999,-0.0145730058670233));
#28871=CARTESIAN_POINT('Ctrl Pts',(-0.00150000000000005,-0.02325,-0.0145730058670132));
#28872=CARTESIAN_POINT('Ctrl Pts',(-0.00150000000000005,-0.0234384855154046,
-0.0145730058670132));
#28873=CARTESIAN_POINT('Ctrl Pts',(-0.00146230406011339,-0.0236394436977337,
-0.0145770395249265));
#28874=CARTESIAN_POINT('Ctrl Pts',(-0.0013091826207289,-0.0240089732900866,
-0.0145915885123659));
#28875=CARTESIAN_POINT('Ctrl Pts',(-0.00119376432903972,-0.02417755601452,
-0.0146018915486848));
#28876=CARTESIAN_POINT('Ctrl Pts',(-0.000927556512672313,-0.0244437638308874,
-0.0146212157105806));
#28877=CARTESIAN_POINT('Ctrl Pts',(-0.000758973570028516,-0.0245591825115081,
-0.0146314951324582));
#28878=CARTESIAN_POINT('Ctrl Pts',(-0.000389443245922634,-0.0247123042405513,
-0.0146459900535486));
#28879=CARTESIAN_POINT('Ctrl Pts',(-0.000188484809983483,-0.02475,-0.0146500000000001));
#28880=CARTESIAN_POINT('Ctrl Pts',(0.000188484809983392,-0.02475,-0.0146500000000001));
#28881=CARTESIAN_POINT('Ctrl Pts',(0.000389443245922547,-0.0247123042405513,
-0.0146459900535486));
#28882=CARTESIAN_POINT('Ctrl Pts',(0.000758973570028428,-0.0245591825115081,
-0.0146314951324582));
#28883=CARTESIAN_POINT('Ctrl Pts',(0.000927556512672222,-0.0244437638308874,
-0.0146212157105806));
#28884=CARTESIAN_POINT('Ctrl Pts',(0.00119376432903963,-0.02417755601452,
-0.0146018915486848));
#28885=CARTESIAN_POINT('Ctrl Pts',(0.00130918262072881,-0.0240089732900866,
-0.0145915885123659));
#28886=CARTESIAN_POINT('Ctrl Pts',(0.00146230406011329,-0.0236394436977337,
-0.0145770395249265));
#28887=CARTESIAN_POINT('Ctrl Pts',(0.00149999999999995,-0.0234384855154046,
-0.0145730058670132));
#28888=CARTESIAN_POINT('Ctrl Pts',(0.00149999999999995,-0.02325,-0.0145730058670132));
#28889=CARTESIAN_POINT('Origin',(0.00463991534334936,-0.00365,-0.0131027167261814));
#28890=CARTESIAN_POINT('',(0.00463991534334936,-0.02475,-0.0131027167261814));
#28891=CARTESIAN_POINT('',(0.00231995767168467,-0.02475000000001,-0.00655135836310071));
#28892=CARTESIAN_POINT('',(0.00463991534334936,-0.00815,-0.0131027167261814));
#28893=CARTESIAN_POINT('',(0.00231995767168467,-0.00814999999999,-0.00655135836310071));
#28894=CARTESIAN_POINT('',(0.00463991534335936,-0.00364999999999,-0.0131027167261914));
#28895=CARTESIAN_POINT('Origin',(0.000905995435036393,-0.0059,-0.00705206865194137));
#28896=CARTESIAN_POINT('',(0.00170263522945395,-0.00365,-0.0137953265012259));
#28897=CARTESIAN_POINT('',(-0.000507966801611876,-0.00364999999999,-0.00755277894080202));
#28898=CARTESIAN_POINT('Origin',(-4.56515315114362E-17,-0.00814999999999,
-6.77116287837691E-17));
#28899=CARTESIAN_POINT('Origin',(-4.56515315114362E-17,-0.00365,-6.77116287837691E-17));
#28900=CARTESIAN_POINT('',(-0.00170263522945404,-0.00365,-0.0137953265012259));
#28901=CARTESIAN_POINT('',(0.000382789229399116,-0.00364999999999,-0.00790626949996159));
#28902=CARTESIAN_POINT('Origin',(-4.56515315114362E-17,-0.00364999999999,
-6.77116287837691E-17));
#28903=CARTESIAN_POINT('Origin',(-0.00103117300724916,-0.0059,-0.00740555921110094));
#28904=CARTESIAN_POINT('',(-0.00463991534334947,-0.00815,-0.0131027167261814));
#28905=CARTESIAN_POINT('Origin',(-4.56515315114362E-17,-0.00814999999999,
-6.77116287837691E-17));
#28906=CARTESIAN_POINT('',(-0.00244513524389743,-0.00814999999999,-0.00690484892226028));
#28907=CARTESIAN_POINT('Origin',(-0.0048902704877748,-0.00365,-0.0138096978445005));
#28908=CARTESIAN_POINT('',(-0.00463991534334947,-0.02475,-0.0131027167261814));
#28909=CARTESIAN_POINT('',(-0.00244513524389742,-0.02475000000001,-0.00690484892226028));
#28910=CARTESIAN_POINT('',(-0.00463991534335947,-0.00364999999999,-0.0131027167261914));
#28911=CARTESIAN_POINT('Origin',(-0.00103117300724916,-0.027,-0.00740555921110094));
#28912=CARTESIAN_POINT('',(-0.00170263522945404,-0.02925,-0.0137953265012259));
#28913=CARTESIAN_POINT('',(0.000382789229399114,-0.02925000000001,-0.00790626949996159));
#28914=CARTESIAN_POINT('Origin',(-4.56515315114362E-17,-0.02475000000001,
-6.77116287837691E-17));
#28915=CARTESIAN_POINT('Origin',(-4.56515315114362E-17,-0.00365,-6.77116287837691E-17));
#28916=CARTESIAN_POINT('',(0.00170263522945395,-0.02925,-0.0137953265012259));
#28917=CARTESIAN_POINT('Origin',(-4.56515315114362E-17,-0.02475000000001,
-6.77116287837691E-17));
#28918=CARTESIAN_POINT('Origin',(-4.56515315114362E-17,-0.02925000000001,
-6.77116287837691E-17));
#28919=CARTESIAN_POINT('Origin',(-4.56515315114362E-17,-0.02925,-6.77116287837691E-17));
#28920=CARTESIAN_POINT('',(-0.000507966801611876,-0.02925000000001,-0.00755277894080202));
#28921=CARTESIAN_POINT('Origin',(0.000905995435036393,-0.027,-0.00705206865194137));
#28922=CARTESIAN_POINT('Origin',(-0.00150000000000005,-0.00965,-0.0184));
#28923=CARTESIAN_POINT('',(-0.00150000000000005,-0.00965,-0.0184));
#28924=CARTESIAN_POINT('',(-0.00150000000001004,-0.00964999999999,-0.0184000000000101));
#28925=CARTESIAN_POINT('',(-0.00150000000000005,-0.02325,-0.0184));
#28926=CARTESIAN_POINT('',(-0.00150000000001003,-0.00964999999999,-0.0184000000000101));
#28927=CARTESIAN_POINT('',(-0.00150000000001004,-0.02325000000001,-0.0184000000000101));
#28928=CARTESIAN_POINT('Origin',(-4.56515315114362E-17,-0.00965,-0.0184));
#28929=CARTESIAN_POINT('',(0.00149999999999995,-0.00965,-0.0184));
#28930=CARTESIAN_POINT('',(0.00150000000000995,-0.00964999999999,-0.0184000000000101));
#28931=CARTESIAN_POINT('Origin',(-4.56515315114362E-17,-0.00964999999999,
-0.0184000000000101));
#28932=CARTESIAN_POINT('Origin',(-4.56515315114362E-17,-0.02325,-0.0184));
#28933=CARTESIAN_POINT('',(0.00149999999999995,-0.02325,-0.0184));
#28934=CARTESIAN_POINT('Origin',(-4.56515315114362E-17,-0.02325000000001,
-0.0184000000000101));
#28935=CARTESIAN_POINT('',(0.00150000000000995,-0.02325000000001,-0.0184000000000101));
#28936=CARTESIAN_POINT('Origin',(0.00149999999999995,-0.02325,-0.0184));
#28937=CARTESIAN_POINT('',(0.00150000000000995,-0.02325000000001,-0.0184000000000101));
#28938=CARTESIAN_POINT('Origin',(-4.56515315114362E-17,-0.00365,-6.77116287837691E-17));
#28939=CARTESIAN_POINT('',(-0.00888108833605081,-0.02925,-0.0116511274118544));
#28940=CARTESIAN_POINT('',(-0.00630698756824158,-0.02475,-0.0132228744157256));
#28941=CARTESIAN_POINT('Origin',(-4.56515315114362E-17,-0.02475000000001,
-6.77116287837691E-17));
#28942=CARTESIAN_POINT('',(-0.0116511274118543,-0.02925,-0.00888108833605082));
#28943=CARTESIAN_POINT('Origin',(-4.56515315114362E-17,-0.02925000000001,
-6.77116287837691E-17));
#28944=CARTESIAN_POINT('',(-0.0132228744157255,-0.02475,-0.00630698756824159));
#28945=CARTESIAN_POINT('Origin',(-4.56515315114362E-17,-0.02475000000001,
-6.77116287837691E-17));
#28946=CARTESIAN_POINT('',(-0.0132228744157255,-0.00815,-0.00630698756824159));
#28947=CARTESIAN_POINT('',(-0.0132228744157355,-0.00364999999999,-0.00630698756825159));
#28948=CARTESIAN_POINT('',(-0.0116511274118543,-0.00365,-0.00888108833605082));
#28949=CARTESIAN_POINT('Origin',(-4.56515315114362E-17,-0.00814999999999,
-6.77116287837691E-17));
#28950=CARTESIAN_POINT('',(-0.00888108833605081,-0.00365,-0.0116511274118544));
#28951=CARTESIAN_POINT('Origin',(-4.56515315114362E-17,-0.00364999999999,
-6.77116287837691E-17));
#28952=CARTESIAN_POINT('',(-0.00630698756824158,-0.00815,-0.0132228744157256));
#28953=CARTESIAN_POINT('Origin',(-4.56515315114362E-17,-0.00814999999999,
-6.77116287837691E-17));
#28954=CARTESIAN_POINT('',(-0.00630698756825158,-0.00364999999999,-0.0132228744157356));
#28955=CARTESIAN_POINT('',(-0.00924401109905658,-0.02325,-0.0113653314426163));
#28956=CARTESIAN_POINT('',(-0.00924401109905658,-0.00965,-0.0113653314426163));
#28957=CARTESIAN_POINT('',(-0.00924401109906658,-0.00364999999999,-0.0113653314426263));
#28958=CARTESIAN_POINT('',(-0.0113653314426162,-0.00965,-0.0092440110990566));
#28959=CARTESIAN_POINT('Ctrl Pts',(-0.00924401109905653,-0.00965,-0.0113653314426163));
#28960=CARTESIAN_POINT('Ctrl Pts',(-0.00924401109905653,-0.00946151448459537,
-0.0113653314426163));
#28961=CARTESIAN_POINT('Ctrl Pts',(-0.00927351838063707,-0.00926055630226628,
-0.0113415286147627));
#28962=CARTESIAN_POINT('Ctrl Pts',(-0.00939207927644867,-0.00889102670991339,
-0.0112435430943067));
#28963=CARTESIAN_POINT('Ctrl Pts',(-0.00948097768002294,-0.00872244398548004,
-0.0111692153844282));
#28964=CARTESIAN_POINT('Ctrl Pts',(-0.00968287927809846,-0.00845623616911263,
-0.0109946422781872));
#28965=CARTESIAN_POINT('Ctrl Pts',(-0.00980935406895063,-0.00834081748849188,
-0.0108827047851677));
#28966=CARTESIAN_POINT('Ctrl Pts',(-0.0100809009239757,-0.00818769575944871,
-0.0106316568441342));
#28967=CARTESIAN_POINT('Ctrl Pts',(-0.010225835457093,-0.00815,-0.010492393231673));
#28968=CARTESIAN_POINT('Ctrl Pts',(-0.0104923932316729,-0.00815,-0.0102258354570931));
#28969=CARTESIAN_POINT('Ctrl Pts',(-0.0106316568441341,-0.00818769575944871,
-0.0100809009239758));
#28970=CARTESIAN_POINT('Ctrl Pts',(-0.0108827047851676,-0.00834081748849188,
-0.00980935406895074));
#28971=CARTESIAN_POINT('Ctrl Pts',(-0.0109946422781871,-0.00845623616911263,
-0.00968287927809856));
#28972=CARTESIAN_POINT('Ctrl Pts',(-0.0111692153844281,-0.00872244398548004,
-0.00948097768002304));
#28973=CARTESIAN_POINT('Ctrl Pts',(-0.0112435430943066,-0.00889102670991339,
-0.00939207927644877));
#28974=CARTESIAN_POINT('Ctrl Pts',(-0.0113415286147626,-0.00926055630226628,
-0.00927351838063717));
#28975=CARTESIAN_POINT('Ctrl Pts',(-0.0113653314426162,-0.00946151448459537,
-0.00924401109905664));
#28976=CARTESIAN_POINT('Ctrl Pts',(-0.0113653314426162,-0.00965,-0.00924401109905664));
#28977=CARTESIAN_POINT('',(-0.0113653314426162,-0.02325,-0.0092440110990566));
#28978=CARTESIAN_POINT('',(-0.0113653314426262,-0.00364999999999,-0.0092440110990666));
#28979=CARTESIAN_POINT('Ctrl Pts',(-0.0113653314426162,-0.02325,-0.00924401109905664));
#28980=CARTESIAN_POINT('Ctrl Pts',(-0.0113653314426162,-0.0234384855154046,
-0.00924401109905664));
#28981=CARTESIAN_POINT('Ctrl Pts',(-0.0113415286147626,-0.0236394436977337,
-0.00927351838063718));
#28982=CARTESIAN_POINT('Ctrl Pts',(-0.0112435430943066,-0.0240089732900866,
-0.00939207927644877));
#28983=CARTESIAN_POINT('Ctrl Pts',(-0.0111692153844281,-0.02417755601452,
-0.00948097768002304));
#28984=CARTESIAN_POINT('Ctrl Pts',(-0.0109946422781871,-0.0244437638308874,
-0.00968287927809855));
#28985=CARTESIAN_POINT('Ctrl Pts',(-0.0108827047851676,-0.0245591825115081,
-0.00980935406895074));
#28986=CARTESIAN_POINT('Ctrl Pts',(-0.0106316568441341,-0.0247123042405513,
-0.0100809009239758));
#28987=CARTESIAN_POINT('Ctrl Pts',(-0.0104923932316729,-0.02475,-0.0102258354570931));
#28988=CARTESIAN_POINT('Ctrl Pts',(-0.010225835457093,-0.02475,-0.010492393231673));
#28989=CARTESIAN_POINT('Ctrl Pts',(-0.0100809009239757,-0.0247123042405513,
-0.0106316568441342));
#28990=CARTESIAN_POINT('Ctrl Pts',(-0.00980935406895064,-0.0245591825115081,
-0.0108827047851677));
#28991=CARTESIAN_POINT('Ctrl Pts',(-0.00968287927809846,-0.0244437638308874,
-0.0109946422781872));
#28992=CARTESIAN_POINT('Ctrl Pts',(-0.00948097768002294,-0.02417755601452,
-0.0111692153844282));
#28993=CARTESIAN_POINT('Ctrl Pts',(-0.00939207927644866,-0.0240089732900866,
-0.0112435430943067));
#28994=CARTESIAN_POINT('Ctrl Pts',(-0.00927351838063707,-0.0236394436977337,
-0.0113415286147627));
#28995=CARTESIAN_POINT('Ctrl Pts',(-0.00924401109905653,-0.0234384855154046,
-0.0113653314426163));
#28996=CARTESIAN_POINT('Ctrl Pts',(-0.00924401109905653,-0.02325,-0.0113653314426163));
#28997=CARTESIAN_POINT('Origin',(-0.00598410424563536,-0.00365,-0.0125459354524632));
#28998=CARTESIAN_POINT('',(-0.00598410424563536,-0.02475,-0.0125459354524632));
#28999=CARTESIAN_POINT('',(-0.0029920521228277,-0.02475000000001,-0.0062729677262416));
#29000=CARTESIAN_POINT('',(-0.00598410424563536,-0.00815,-0.0125459354524632));
#29001=CARTESIAN_POINT('',(-0.0029920521228277,-0.00814999999999,-0.0062729677262416));
#29002=CARTESIAN_POINT('',(-0.00598410424564536,-0.00364999999999,-0.0125459354524732));
#29003=CARTESIAN_POINT('Origin',(-0.00434593004934249,-0.0059,-0.00562720108101916));
#29004=CARTESIAN_POINT('',(-0.00855082400106526,-0.00365,-0.0109587138343334));
#29005=CARTESIAN_POINT('',(-0.00569980797587729,-0.00364999999999,-0.00498143443581672));
#29006=CARTESIAN_POINT('Origin',(-4.56515315114362E-17,-0.00814999999999,
-6.77116287837691E-17));
#29007=CARTESIAN_POINT('Origin',(-4.56515315114362E-17,-0.00365,-6.77116287837691E-17));
#29008=CARTESIAN_POINT('',(-0.0109587138343333,-0.00365,-0.00855082400106528));
#29009=CARTESIAN_POINT('',(-0.0053199039174479,-0.00364999999999,-0.00586124963718042));
#29010=CARTESIAN_POINT('Origin',(-4.56515315114362E-17,-0.00364999999999,
-6.77116287837691E-17));
#29011=CARTESIAN_POINT('Origin',(-0.00596567056265034,-0.0059,-0.00450737171064562));
#29012=CARTESIAN_POINT('',(-0.0125459354524631,-0.00815,-0.00598410424563537));
#29013=CARTESIAN_POINT('Origin',(-4.56515315114362E-17,-0.00814999999999,
-6.77116287837691E-17));
#29014=CARTESIAN_POINT('',(-0.00661143720787278,-0.00814999999999,-0.00315349378413083));
#29015=CARTESIAN_POINT('Origin',(-0.0132228744157255,-0.00365,-0.00630698756824159));
#29016=CARTESIAN_POINT('',(-0.0125459354524631,-0.02475,-0.00598410424563537));
#29017=CARTESIAN_POINT('',(-0.00661143720787278,-0.02475000000001,-0.00315349378413083));
#29018=CARTESIAN_POINT('',(-0.0125459354524731,-0.00364999999999,-0.00598410424564537));
#29019=CARTESIAN_POINT('Origin',(-0.00596567056265034,-0.027,-0.00450737171064562));
#29020=CARTESIAN_POINT('',(-0.0109587138343333,-0.02925,-0.00855082400106528));
#29021=CARTESIAN_POINT('',(-0.0053199039174479,-0.02925000000001,-0.00586124963718041));
#29022=CARTESIAN_POINT('Origin',(-4.56515315114362E-17,-0.02475000000001,
-6.77116287837691E-17));
#29023=CARTESIAN_POINT('Origin',(-4.56515315114362E-17,-0.00365,-6.77116287837691E-17));
#29024=CARTESIAN_POINT('',(-0.00855082400106526,-0.02925,-0.0109587138343334));
#29025=CARTESIAN_POINT('Origin',(-4.56515315114362E-17,-0.02475000000001,
-6.77116287837691E-17));
#29026=CARTESIAN_POINT('Origin',(-4.56515315114362E-17,-0.02925000000001,
-6.77116287837691E-17));
#29027=CARTESIAN_POINT('Origin',(-4.56515315114362E-17,-0.02925,-6.77116287837691E-17));
#29028=CARTESIAN_POINT('',(-0.00569980797587729,-0.02925000000001,-0.00498143443581672));
#29029=CARTESIAN_POINT('Origin',(-0.00434593004934249,-0.027,-0.00562720108101916));
#29030=CARTESIAN_POINT('Origin',(-0.0140714249456123,-0.00965,-0.0119501046020528));
#29031=CARTESIAN_POINT('',(-0.0140714249456123,-0.00965,-0.0119501046020528));
#29032=CARTESIAN_POINT('',(-0.0140714249456223,-0.00964999999999,-0.0119501046020628));
#29033=CARTESIAN_POINT('',(-0.0140714249456123,-0.02325,-0.0119501046020528));
#29034=CARTESIAN_POINT('',(-0.0140714249456223,-0.00964999999999,-0.0119501046020628));
#29035=CARTESIAN_POINT('',(-0.0140714249456223,-0.02325000000001,-0.0119501046020628));
#29036=CARTESIAN_POINT('Origin',(-0.0130107647738325,-0.00965,-0.0130107647738326));
#29037=CARTESIAN_POINT('',(-0.0119501046020527,-0.00965,-0.0140714249456124));
#29038=CARTESIAN_POINT('',(-0.0119501046020627,-0.00964999999999,-0.0140714249456224));
#29039=CARTESIAN_POINT('Origin',(-0.0130107647738425,-0.00964999999999,
-0.0130107647738426));
#29040=CARTESIAN_POINT('Origin',(-0.0130107647738325,-0.02325,-0.0130107647738326));
#29041=CARTESIAN_POINT('',(-0.0119501046020527,-0.02325,-0.0140714249456124));
#29042=CARTESIAN_POINT('Origin',(-0.0130107647738425,-0.02325000000001,
-0.0130107647738426));
#29043=CARTESIAN_POINT('',(-0.0119501046020627,-0.02325000000001,-0.0140714249456224));
#29044=CARTESIAN_POINT('Origin',(-0.0119501046020527,-0.02325,-0.0140714249456124));
#29045=CARTESIAN_POINT('',(-0.0119501046020627,-0.02325000000001,-0.0140714249456224));
#29046=CARTESIAN_POINT('Origin',(-4.56515315114362E-17,-0.00365,-6.77116287837691E-17));
#29047=CARTESIAN_POINT('',(-0.0145184689881289,-0.02925,-0.00195871341465249));
#29048=CARTESIAN_POINT('',(-0.0138096978445004,-0.02475,-0.00489027048777481));
#29049=CARTESIAN_POINT('Origin',(-4.56515315114362E-17,-0.02475000000001,
-6.77116287837691E-17));
#29050=CARTESIAN_POINT('',(-0.0145184689881289,-0.02925,0.00195871341465236));
#29051=CARTESIAN_POINT('Origin',(-4.56515315114362E-17,-0.02925000000001,
-6.77116287837691E-17));
#29052=CARTESIAN_POINT('',(-0.0138096978445004,-0.02475,0.00489027048777468));
#29053=CARTESIAN_POINT('Origin',(-4.56515315114362E-17,-0.02475000000001,
-6.77116287837691E-17));
#29054=CARTESIAN_POINT('',(-0.0138096978445004,-0.00815,0.00489027048777468));
#29055=CARTESIAN_POINT('',(-0.0138096978445104,-0.00364999999999,0.00489027048778468));
#29056=CARTESIAN_POINT('',(-0.0145184689881289,-0.00365,0.00195871341465235));
#29057=CARTESIAN_POINT('Origin',(-4.56515315114362E-17,-0.00814999999999,
-6.77116287837691E-17));
#29058=CARTESIAN_POINT('',(-0.0145184689881289,-0.00365,-0.00195871341465249));
#29059=CARTESIAN_POINT('Origin',(-4.56515315114362E-17,-0.00364999999999,
-6.77116287837691E-17));
#29060=CARTESIAN_POINT('',(-0.0138096978445004,-0.00815,-0.00489027048777481));
#29061=CARTESIAN_POINT('Origin',(-4.56515315114362E-17,-0.00814999999999,
-6.77116287837691E-17));
#29062=CARTESIAN_POINT('',(-0.0138096978445104,-0.00364999999999,-0.00489027048778481));
#29063=CARTESIAN_POINT('',(-0.0145730058670132,-0.02325,-0.00150000000000007));
#29064=CARTESIAN_POINT('',(-0.0145730058670132,-0.00965,-0.00150000000000007));
#29065=CARTESIAN_POINT('',(-0.0145730058670232,-0.00364999999999,-0.00150000000001007));
#29066=CARTESIAN_POINT('',(-0.0145730058670132,-0.00965,0.00149999999999993));
#29067=CARTESIAN_POINT('Ctrl Pts',(-0.0145730058670132,-0.00965,-0.00150000000000007));
#29068=CARTESIAN_POINT('Ctrl Pts',(-0.0145730058670132,-0.00946151448459537,
-0.00150000000000007));
#29069=CARTESIAN_POINT('Ctrl Pts',(-0.0145770395249265,-0.00926055630226629,
-0.00146230406011341));
#29070=CARTESIAN_POINT('Ctrl Pts',(-0.0145915885123659,-0.00889102670991339,
-0.00130918262072893));
#29071=CARTESIAN_POINT('Ctrl Pts',(-0.0146018915486848,-0.00872244398548004,
-0.00119376432903975));
#29072=CARTESIAN_POINT('Ctrl Pts',(-0.0146212157105805,-0.00845623616911263,
-0.000927556512672337));
#29073=CARTESIAN_POINT('Ctrl Pts',(-0.0146314951324582,-0.00834081748849188,
-0.000758973570028542));
#29074=CARTESIAN_POINT('Ctrl Pts',(-0.0146459900535486,-0.00818769575944871,
-0.000389443245922659));
#29075=CARTESIAN_POINT('Ctrl Pts',(-0.01465,-0.00815,-0.000188484809983507));
#29076=CARTESIAN_POINT('Ctrl Pts',(-0.01465,-0.00815,0.000188484809983367));
#29077=CARTESIAN_POINT('Ctrl Pts',(-0.0146459900535486,-0.00818769575944871,
0.000389443245922518));
#29078=CARTESIAN_POINT('Ctrl Pts',(-0.0146314951324582,-0.00834081748849188,
0.000758973570028401));
#29079=CARTESIAN_POINT('Ctrl Pts',(-0.0146212157105805,-0.00845623616911263,
0.000927556512672196));
#29080=CARTESIAN_POINT('Ctrl Pts',(-0.0146018915486848,-0.00872244398548004,
0.00119376432903961));
#29081=CARTESIAN_POINT('Ctrl Pts',(-0.0145915885123659,-0.00889102670991339,
0.00130918262072879));
#29082=CARTESIAN_POINT('Ctrl Pts',(-0.0145770395249265,-0.00926055630226629,
0.00146230406011327));
#29083=CARTESIAN_POINT('Ctrl Pts',(-0.0145730058670132,-0.00946151448459537,
0.00149999999999993));
#29084=CARTESIAN_POINT('Ctrl Pts',(-0.0145730058670132,-0.00965,0.00149999999999993));
#29085=CARTESIAN_POINT('',(-0.0145730058670132,-0.02325,0.00149999999999993));
#29086=CARTESIAN_POINT('',(-0.0145730058670232,-0.00364999999999,0.00150000000000993));
#29087=CARTESIAN_POINT('Ctrl Pts',(-0.0145730058670132,-0.02325,0.00149999999999993));
#29088=CARTESIAN_POINT('Ctrl Pts',(-0.0145730058670132,-0.0234384855154046,
0.00149999999999993));
#29089=CARTESIAN_POINT('Ctrl Pts',(-0.0145770395249265,-0.0236394436977337,
0.00146230406011327));
#29090=CARTESIAN_POINT('Ctrl Pts',(-0.0145915885123659,-0.0240089732900866,
0.00130918262072879));
#29091=CARTESIAN_POINT('Ctrl Pts',(-0.0146018915486848,-0.02417755601452,
0.00119376432903961));
#29092=CARTESIAN_POINT('Ctrl Pts',(-0.0146212157105805,-0.0244437638308874,
0.000927556512672197));
#29093=CARTESIAN_POINT('Ctrl Pts',(-0.0146314951324582,-0.0245591825115081,
0.0007589735700284));
#29094=CARTESIAN_POINT('Ctrl Pts',(-0.0146459900535486,-0.0247123042405513,
0.000389443245922519));
#29095=CARTESIAN_POINT('Ctrl Pts',(-0.01465,-0.02475,0.000188484809983366));
#29096=CARTESIAN_POINT('Ctrl Pts',(-0.01465,-0.02475,-0.000188484809983508));
#29097=CARTESIAN_POINT('Ctrl Pts',(-0.0146459900535486,-0.0247123042405513,
-0.000389443245922663));
#29098=CARTESIAN_POINT('Ctrl Pts',(-0.0146314951324582,-0.0245591825115081,
-0.000758973570028544));
#29099=CARTESIAN_POINT('Ctrl Pts',(-0.0146212157105805,-0.0244437638308874,
-0.000927556512672338));
#29100=CARTESIAN_POINT('Ctrl Pts',(-0.0146018915486848,-0.02417755601452,
-0.00119376432903975));
#29101=CARTESIAN_POINT('Ctrl Pts',(-0.0145915885123659,-0.0240089732900866,
-0.00130918262072893));
#29102=CARTESIAN_POINT('Ctrl Pts',(-0.0145770395249265,-0.0236394436977337,
-0.00146230406011341));
#29103=CARTESIAN_POINT('Ctrl Pts',(-0.0145730058670132,-0.0234384855154046,
-0.00150000000000007));
#29104=CARTESIAN_POINT('Ctrl Pts',(-0.0145730058670132,-0.02325,-0.00150000000000007));
#29105=CARTESIAN_POINT('Origin',(-0.0131027167261813,-0.00365,-0.00463991534334948));
#29106=CARTESIAN_POINT('',(-0.0131027167261813,-0.02475,-0.00463991534334948));
#29107=CARTESIAN_POINT('',(-0.00655135836310069,-0.02475000000001,-0.00231995767168478));
#29108=CARTESIAN_POINT('',(-0.0131027167261813,-0.00815,-0.00463991534334948));
#29109=CARTESIAN_POINT('',(-0.00655135836310069,-0.00814999999999,-0.00231995767168478));
#29110=CARTESIAN_POINT('',(-0.0131027167261913,-0.00364999999999,-0.00463991534335948));
#29111=CARTESIAN_POINT('Origin',(-0.00705206865194135,-0.0059,-0.000905995435036507));
#29112=CARTESIAN_POINT('',(-0.0137953265012258,-0.00365,-0.00170263522945406));
#29113=CARTESIAN_POINT('',(-0.007552778940802,-0.00364999999999,0.000507966801611762));
#29114=CARTESIAN_POINT('Origin',(-4.56515315114362E-17,-0.00814999999999,
-6.77116287837691E-17));
#29115=CARTESIAN_POINT('Origin',(-4.56515315114362E-17,-0.00365,-6.77116287837691E-17));
#29116=CARTESIAN_POINT('',(-0.0137953265012258,-0.00365,0.00170263522945392));
#29117=CARTESIAN_POINT('',(-0.00790626949996156,-0.00364999999999,-0.00038278922939923));
#29118=CARTESIAN_POINT('Origin',(-4.56515315114362E-17,-0.00364999999999,
-6.77116287837691E-17));
#29119=CARTESIAN_POINT('Origin',(-0.00740555921110092,-0.0059,0.00103117300724904));
#29120=CARTESIAN_POINT('',(-0.0131027167261813,-0.00815,0.00463991534334935));
#29121=CARTESIAN_POINT('Origin',(-4.56515315114362E-17,-0.00814999999999,
-6.77116287837691E-17));
#29122=CARTESIAN_POINT('',(-0.00690484892226026,-0.00814999999999,0.00244513524389732));
#29123=CARTESIAN_POINT('Origin',(-0.0138096978445004,-0.00365,0.00489027048777468));
#29124=CARTESIAN_POINT('',(-0.0131027167261813,-0.02475,0.00463991534334935));
#29125=CARTESIAN_POINT('',(-0.00690484892226026,-0.02475000000001,0.0024451352438973));
#29126=CARTESIAN_POINT('',(-0.0131027167261913,-0.00364999999999,0.00463991534335935));
#29127=CARTESIAN_POINT('Origin',(-0.00740555921110092,-0.027,0.00103117300724904));
#29128=CARTESIAN_POINT('',(-0.0137953265012258,-0.02925,0.00170263522945392));
#29129=CARTESIAN_POINT('',(-0.00790626949996156,-0.02925000000001,-0.000382789229399229));
#29130=CARTESIAN_POINT('Origin',(-4.56515315114362E-17,-0.02475000000001,
-6.77116287837691E-17));
#29131=CARTESIAN_POINT('Origin',(-4.56515315114362E-17,-0.00365,-6.77116287837691E-17));
#29132=CARTESIAN_POINT('',(-0.0137953265012258,-0.02925,-0.00170263522945406));
#29133=CARTESIAN_POINT('Origin',(-4.56515315114362E-17,-0.02475000000001,
-6.77116287837691E-17));
#29134=CARTESIAN_POINT('Origin',(-4.56515315114362E-17,-0.02925000000001,
-6.77116287837691E-17));
#29135=CARTESIAN_POINT('Origin',(-4.56515315114362E-17,-0.02925,-6.77116287837691E-17));
#29136=CARTESIAN_POINT('',(-0.007552778940802,-0.02925000000001,0.000507966801611762));
#29137=CARTESIAN_POINT('Origin',(-0.00705206865194135,-0.027,-0.000905995435036507));
#29138=CARTESIAN_POINT('Origin',(-0.0184,-0.00965,0.00149999999999993));
#29139=CARTESIAN_POINT('',(-0.0184,-0.00965,0.00149999999999993));
#29140=CARTESIAN_POINT('',(-0.0184000000000101,-0.00964999999999,0.00150000000000993));
#29141=CARTESIAN_POINT('',(-0.0184,-0.02325,0.00149999999999993));
#29142=CARTESIAN_POINT('',(-0.0184000000000101,-0.00964999999999,0.00150000000000993));
#29143=CARTESIAN_POINT('',(-0.0184000000000101,-0.02325000000001,0.00150000000000993));
#29144=CARTESIAN_POINT('Origin',(-0.0184,-0.00965,-7.10422978576446E-17));
#29145=CARTESIAN_POINT('',(-0.0184,-0.00965,-0.00150000000000007));
#29146=CARTESIAN_POINT('',(-0.0184000000000101,-0.00964999999999,-0.00150000000001007));
#29147=CARTESIAN_POINT('Origin',(-0.0184000000000101,-0.00964999999999,
-1.00710422978576E-14));
#29148=CARTESIAN_POINT('Origin',(-0.0184,-0.02325,-7.10422978576446E-17));
#29149=CARTESIAN_POINT('',(-0.0184,-0.02325,-0.00150000000000007));
#29150=CARTESIAN_POINT('Origin',(-0.0184000000000101,-0.02325000000001,
-1.00710422978576E-14));
#29151=CARTESIAN_POINT('',(-0.0184000000000101,-0.02325000000001,-0.00150000000001008));
#29152=CARTESIAN_POINT('Origin',(-0.0184,-0.02325,-0.00150000000000007));
#29153=CARTESIAN_POINT('',(-0.0184000000000101,-0.02325000000001,-0.00150000000001007));
#29154=CARTESIAN_POINT('Origin',(-4.56515315114362E-17,-0.00365,-6.77116287837691E-17));
#29155=CARTESIAN_POINT('',(-0.0116511274118543,-0.02925,0.00888108833605068));
#29156=CARTESIAN_POINT('',(-0.0132228744157255,-0.02475,0.00630698756824146));
#29157=CARTESIAN_POINT('Origin',(-4.56515315114362E-17,-0.02475000000001,
-6.77116287837691E-17));
#29158=CARTESIAN_POINT('',(-0.0088810883360508,-0.02925,0.0116511274118542));
#29159=CARTESIAN_POINT('Origin',(-4.56515315114362E-17,-0.02925000000001,
-6.77116287837691E-17));
#29160=CARTESIAN_POINT('',(-0.00630698756824158,-0.02475,0.0132228744157254));
#29161=CARTESIAN_POINT('Origin',(-4.56515315114362E-17,-0.02475000000001,
-6.77116287837691E-17));
#29162=CARTESIAN_POINT('',(-0.00630698756824158,-0.00815,0.0132228744157254));
#29163=CARTESIAN_POINT('',(-0.00630698756825158,-0.00364999999999,0.0132228744157354));
#29164=CARTESIAN_POINT('',(-0.00888108833605081,-0.00365,0.0116511274118542));
#29165=CARTESIAN_POINT('Origin',(-4.56515315114362E-17,-0.00814999999999,
-6.77116287837691E-17));
#29166=CARTESIAN_POINT('',(-0.0116511274118543,-0.00365,0.00888108833605068));
#29167=CARTESIAN_POINT('Origin',(-4.56515315114362E-17,-0.00364999999999,
-6.77116287837691E-17));
#29168=CARTESIAN_POINT('',(-0.0132228744157255,-0.00815,0.00630698756824146));
#29169=CARTESIAN_POINT('Origin',(-4.56515315114362E-17,-0.00814999999999,
-6.77116287837691E-17));
#29170=CARTESIAN_POINT('',(-0.0132228744157355,-0.00364999999999,0.00630698756825146));
#29171=CARTESIAN_POINT('',(-0.0113653314426162,-0.02325,0.00924401109905646));
#29172=CARTESIAN_POINT('',(-0.0113653314426162,-0.00965,0.00924401109905646));
#29173=CARTESIAN_POINT('',(-0.0113653314426262,-0.00364999999999,0.00924401109906646));
#29174=CARTESIAN_POINT('',(-0.00924401109905658,-0.00965,0.0113653314426161));
#29175=CARTESIAN_POINT('Ctrl Pts',(-0.0113653314426162,-0.00965,0.00924401109905647));
#29176=CARTESIAN_POINT('Ctrl Pts',(-0.0113653314426162,-0.00946151448459537,
0.00924401109905647));
#29177=CARTESIAN_POINT('Ctrl Pts',(-0.0113415286147626,-0.00926055630226629,
0.00927351838063701));
#29178=CARTESIAN_POINT('Ctrl Pts',(-0.0112435430943066,-0.00889102670991339,
0.0093920792764486));
#29179=CARTESIAN_POINT('Ctrl Pts',(-0.0111692153844281,-0.00872244398548004,
0.00948097768002287));
#29180=CARTESIAN_POINT('Ctrl Pts',(-0.0109946422781871,-0.00845623616911263,
0.00968287927809839));
#29181=CARTESIAN_POINT('Ctrl Pts',(-0.0108827047851677,-0.00834081748849188,
0.00980935406895057));
#29182=CARTESIAN_POINT('Ctrl Pts',(-0.0106316568441341,-0.00818769575944871,
0.0100809009239757));
#29183=CARTESIAN_POINT('Ctrl Pts',(-0.0104923932316729,-0.00815,0.0102258354570929));
#29184=CARTESIAN_POINT('Ctrl Pts',(-0.010225835457093,-0.00815,0.0104923932316728));
#29185=CARTESIAN_POINT('Ctrl Pts',(-0.0100809009239758,-0.00818769575944871,
0.010631656844134));
#29186=CARTESIAN_POINT('Ctrl Pts',(-0.00980935406895067,-0.00834081748849188,
0.0108827047851676));
#29187=CARTESIAN_POINT('Ctrl Pts',(-0.00968287927809849,-0.00845623616911263,
0.010994642278187));
#29188=CARTESIAN_POINT('Ctrl Pts',(-0.00948097768002297,-0.00872244398548004,
0.011169215384428));
#29189=CARTESIAN_POINT('Ctrl Pts',(-0.0093920792764487,-0.00889102670991339,
0.0112435430943065));
#29190=CARTESIAN_POINT('Ctrl Pts',(-0.0092735183806371,-0.00926055630226629,
0.0113415286147625));
#29191=CARTESIAN_POINT('Ctrl Pts',(-0.00924401109905656,-0.00946151448459537,
0.0113653314426161));
#29192=CARTESIAN_POINT('Ctrl Pts',(-0.00924401109905656,-0.00965,0.0113653314426161));
#29193=CARTESIAN_POINT('',(-0.00924401109905658,-0.02325,0.0113653314426161));
#29194=CARTESIAN_POINT('',(-0.00924401109906658,-0.00364999999999,0.0113653314426261));
#29195=CARTESIAN_POINT('Ctrl Pts',(-0.00924401109905656,-0.02325,0.0113653314426161));
#29196=CARTESIAN_POINT('Ctrl Pts',(-0.00924401109905656,-0.0234384855154046,
0.0113653314426161));
#29197=CARTESIAN_POINT('Ctrl Pts',(-0.0092735183806371,-0.0236394436977337,
0.0113415286147625));
#29198=CARTESIAN_POINT('Ctrl Pts',(-0.0093920792764487,-0.0240089732900866,
0.0112435430943065));
#29199=CARTESIAN_POINT('Ctrl Pts',(-0.00948097768002297,-0.02417755601452,
0.011169215384428));
#29200=CARTESIAN_POINT('Ctrl Pts',(-0.00968287927809848,-0.0244437638308874,
0.010994642278187));
#29201=CARTESIAN_POINT('Ctrl Pts',(-0.00980935406895067,-0.0245591825115081,
0.0108827047851676));
#29202=CARTESIAN_POINT('Ctrl Pts',(-0.0100809009239758,-0.0247123042405513,
0.010631656844134));
#29203=CARTESIAN_POINT('Ctrl Pts',(-0.010225835457093,-0.02475,0.0104923932316728));
#29204=CARTESIAN_POINT('Ctrl Pts',(-0.0104923932316729,-0.02475,0.0102258354570929));
#29205=CARTESIAN_POINT('Ctrl Pts',(-0.0106316568441341,-0.0247123042405513,
0.0100809009239757));
#29206=CARTESIAN_POINT('Ctrl Pts',(-0.0108827047851677,-0.0245591825115081,
0.00980935406895057));
#29207=CARTESIAN_POINT('Ctrl Pts',(-0.0109946422781871,-0.0244437638308874,
0.00968287927809839));
#29208=CARTESIAN_POINT('Ctrl Pts',(-0.0111692153844281,-0.02417755601452,
0.00948097768002287));
#29209=CARTESIAN_POINT('Ctrl Pts',(-0.0112435430943066,-0.0240089732900866,
0.0093920792764486));
#29210=CARTESIAN_POINT('Ctrl Pts',(-0.0113415286147626,-0.0236394436977337,
0.00927351838063701));
#29211=CARTESIAN_POINT('Ctrl Pts',(-0.0113653314426162,-0.0234384855154046,
0.00924401109905647));
#29212=CARTESIAN_POINT('Ctrl Pts',(-0.0113653314426162,-0.02325,0.00924401109905647));
#29213=CARTESIAN_POINT('Origin',(-0.0125459354524631,-0.00365,0.00598410424563523));
#29214=CARTESIAN_POINT('',(-0.0125459354524631,-0.02475,0.00598410424563523));
#29215=CARTESIAN_POINT('',(-0.00627296772624158,-0.02475000000001,0.00299205212282759));
#29216=CARTESIAN_POINT('',(-0.0125459354524631,-0.00815,0.00598410424563523));
#29217=CARTESIAN_POINT('',(-0.00627296772624158,-0.00814999999999,0.00299205212282759));
#29218=CARTESIAN_POINT('',(-0.0125459354524731,-0.00364999999999,0.00598410424564523));
#29219=CARTESIAN_POINT('Origin',(-0.00562720108101914,-0.0059,0.00434593004934238));
#29220=CARTESIAN_POINT('',(-0.0109587138343333,-0.00365,0.00855082400106514));
#29221=CARTESIAN_POINT('',(-0.0049814344358167,-0.00364999999999,0.00569980797587716));
#29222=CARTESIAN_POINT('Origin',(-4.56515315114362E-17,-0.00814999999999,
-6.77116287837691E-17));
#29223=CARTESIAN_POINT('Origin',(-4.56515315114362E-17,-0.00365,-6.77116287837691E-17));
#29224=CARTESIAN_POINT('',(-0.00855082400106526,-0.00365,0.0109587138343332));
#29225=CARTESIAN_POINT('',(-0.0058612496371804,-0.00364999999999,0.00531990391744778));
#29226=CARTESIAN_POINT('Origin',(-4.56515315114362E-17,-0.00364999999999,
-6.77116287837691E-17));
#29227=CARTESIAN_POINT('Origin',(-0.0045073717106456,-0.0059,0.00596567056265022));
#29228=CARTESIAN_POINT('',(-0.00598410424563535,-0.00815,0.012545935452463));
#29229=CARTESIAN_POINT('Origin',(-4.56515315114362E-17,-0.00814999999999,
-6.77116287837691E-17));
#29230=CARTESIAN_POINT('',(-0.00315349378413081,-0.00814999999999,0.00661143720787266));
#29231=CARTESIAN_POINT('Origin',(-0.00630698756824157,-0.00365,0.0132228744157254));
#29232=CARTESIAN_POINT('',(-0.00598410424563535,-0.02475,0.012545935452463));
#29233=CARTESIAN_POINT('',(-0.00315349378413081,-0.02475000000001,0.00661143720787266));
#29234=CARTESIAN_POINT('',(-0.00598410424564535,-0.00364999999999,0.012545935452473));
#29235=CARTESIAN_POINT('Origin',(-0.0045073717106456,-0.027,0.00596567056265022));
#29236=CARTESIAN_POINT('',(-0.00855082400106526,-0.02925,0.0109587138343332));
#29237=CARTESIAN_POINT('',(-0.00586124963718039,-0.02925000000001,0.00531990391744778));
#29238=CARTESIAN_POINT('Origin',(-4.56515315114362E-17,-0.02475000000001,
-6.77116287837691E-17));
#29239=CARTESIAN_POINT('Origin',(-4.56515315114362E-17,-0.00365,-6.77116287837691E-17));
#29240=CARTESIAN_POINT('',(-0.0109587138343333,-0.02925,0.00855082400106514));
#29241=CARTESIAN_POINT('Origin',(-4.56515315114362E-17,-0.02475000000001,
-6.77116287837691E-17));
#29242=CARTESIAN_POINT('Origin',(-4.56515315114362E-17,-0.02925000000001,
-6.77116287837691E-17));
#29243=CARTESIAN_POINT('Origin',(-4.56515315114362E-17,-0.02925,-6.77116287837691E-17));
#29244=CARTESIAN_POINT('',(-0.0049814344358167,-0.02925000000001,0.00569980797587716));
#29245=CARTESIAN_POINT('Origin',(-0.00562720108101914,-0.027,0.00434593004934238));
#29246=CARTESIAN_POINT('Origin',(-0.0119501046020527,-0.00965,0.0140714249456122));
#29247=CARTESIAN_POINT('',(-0.0119501046020527,-0.00965,0.0140714249456122));
#29248=CARTESIAN_POINT('',(-0.0119501046020627,-0.00964999999999,0.0140714249456222));
#29249=CARTESIAN_POINT('',(-0.0119501046020527,-0.02325,0.0140714249456122));
#29250=CARTESIAN_POINT('',(-0.0119501046020627,-0.00964999999999,0.0140714249456222));
#29251=CARTESIAN_POINT('',(-0.0119501046020627,-0.02325000000001,0.0140714249456222));
#29252=CARTESIAN_POINT('Origin',(-0.0130107647738325,-0.00965,0.0130107647738324));
#29253=CARTESIAN_POINT('',(-0.0140714249456123,-0.00965,0.0119501046020526));
#29254=CARTESIAN_POINT('',(-0.0140714249456223,-0.00964999999999,0.0119501046020626));
#29255=CARTESIAN_POINT('Origin',(-0.0130107647738425,-0.00964999999999,
0.0130107647738424));
#29256=CARTESIAN_POINT('Origin',(-0.0130107647738325,-0.02325,0.0130107647738324));
#29257=CARTESIAN_POINT('',(-0.0140714249456123,-0.02325,0.0119501046020526));
#29258=CARTESIAN_POINT('Origin',(-0.0130107647738425,-0.02325000000001,
0.0130107647738424));
#29259=CARTESIAN_POINT('',(-0.0140714249456223,-0.02325000000001,0.0119501046020626));
#29260=CARTESIAN_POINT('Origin',(-0.0140714249456123,-0.02325,0.0119501046020526));
#29261=CARTESIAN_POINT('',(-0.0140714249456223,-0.02325000000001,0.0119501046020626));
#29262=CARTESIAN_POINT('Origin',(-4.56515315114362E-17,-0.00365,-6.77116287837691E-17));
#29263=CARTESIAN_POINT('',(-0.00195871341465247,-0.02925,0.0145184689881288));
#29264=CARTESIAN_POINT('',(-0.00489027048777479,-0.02475,0.0138096978445003));
#29265=CARTESIAN_POINT('Origin',(-4.56515315114362E-17,-0.02475000000001,
-6.77116287837691E-17));
#29266=CARTESIAN_POINT('',(0.00195871341465238,-0.02925,0.0145184689881288));
#29267=CARTESIAN_POINT('Origin',(-4.56515315114362E-17,-0.02925000000001,
-6.77116287837691E-17));
#29268=CARTESIAN_POINT('',(0.0048902704877747,-0.02475,0.0138096978445003));
#29269=CARTESIAN_POINT('Origin',(-4.56515315114362E-17,-0.02475000000001,
-6.77116287837691E-17));
#29270=CARTESIAN_POINT('',(0.0048902704877747,-0.00815,0.0138096978445003));
#29271=CARTESIAN_POINT('',(0.00489027048778471,-0.00364999999999,0.0138096978445103));
#29272=CARTESIAN_POINT('',(0.00195871341465237,-0.00365,0.0145184689881288));
#29273=CARTESIAN_POINT('Origin',(-4.56515315114362E-17,-0.00814999999999,
-6.77116287837691E-17));
#29274=CARTESIAN_POINT('',(-0.00195871341465247,-0.00365,0.0145184689881288));
#29275=CARTESIAN_POINT('Origin',(-4.56515315114362E-17,-0.00364999999999,
-6.77116287837691E-17));
#29276=CARTESIAN_POINT('',(-0.00489027048777479,-0.00815,0.0138096978445003));
#29277=CARTESIAN_POINT('Origin',(-4.56515315114362E-17,-0.00814999999999,
-6.77116287837691E-17));
#29278=CARTESIAN_POINT('',(-0.00489027048778479,-0.00364999999999,0.0138096978445103));
#29279=CARTESIAN_POINT('',(-0.00150000000000005,-0.02325,0.0145730058670131));
#29280=CARTESIAN_POINT('',(-0.00150000000000005,-0.00965,0.0145730058670131));
#29281=CARTESIAN_POINT('',(-0.00150000000001004,-0.00364999999999,0.0145730058670231));
#29282=CARTESIAN_POINT('',(0.00149999999999995,-0.00965,0.0145730058670131));
#29283=CARTESIAN_POINT('Ctrl Pts',(-0.00150000000000005,-0.00965,0.0145730058670131));
#29284=CARTESIAN_POINT('Ctrl Pts',(-0.00150000000000005,-0.00946151448459537,
0.0145730058670131));
#29285=CARTESIAN_POINT('Ctrl Pts',(-0.00146230406011339,-0.00926055630226629,
0.0145770395249264));
#29286=CARTESIAN_POINT('Ctrl Pts',(-0.0013091826207289,-0.00889102670991339,
0.0145915885123658));
#29287=CARTESIAN_POINT('Ctrl Pts',(-0.00119376432903973,-0.00872244398548004,
0.0146018915486846));
#29288=CARTESIAN_POINT('Ctrl Pts',(-0.000927556512672315,-0.00845623616911263,
0.0146212157105804));
#29289=CARTESIAN_POINT('Ctrl Pts',(-0.000758973570028519,-0.00834081748849188,
0.0146314951324581));
#29290=CARTESIAN_POINT('Ctrl Pts',(-0.000389443245922637,-0.00818769575944871,
0.0146459900535485));
#29291=CARTESIAN_POINT('Ctrl Pts',(-0.000188484809983485,-0.00815,0.0146499999999999));
#29292=CARTESIAN_POINT('Ctrl Pts',(0.000188484809983389,-0.00815,0.0146499999999999));
#29293=CARTESIAN_POINT('Ctrl Pts',(0.000389443245922541,-0.00818769575944871,
0.0146459900535485));
#29294=CARTESIAN_POINT('Ctrl Pts',(0.000758973570028423,-0.00834081748849188,
0.0146314951324581));
#29295=CARTESIAN_POINT('Ctrl Pts',(0.000927556512672219,-0.00845623616911263,
0.0146212157105804));
#29296=CARTESIAN_POINT('Ctrl Pts',(0.00119376432903963,-0.00872244398548004,
0.0146018915486846));
#29297=CARTESIAN_POINT('Ctrl Pts',(0.00130918262072881,-0.00889102670991339,
0.0145915885123658));
#29298=CARTESIAN_POINT('Ctrl Pts',(0.00146230406011329,-0.00926055630226629,
0.0145770395249264));
#29299=CARTESIAN_POINT('Ctrl Pts',(0.00149999999999995,-0.00946151448459537,
0.0145730058670131));
#29300=CARTESIAN_POINT('Ctrl Pts',(0.00149999999999995,-0.00965,0.0145730058670131));
#29301=CARTESIAN_POINT('',(0.00149999999999995,-0.02325,0.0145730058670131));
#29302=CARTESIAN_POINT('',(0.00150000000000994,-0.00364999999999,0.0145730058670231));
#29303=CARTESIAN_POINT('Ctrl Pts',(0.00149999999999995,-0.02325,0.0145730058670131));
#29304=CARTESIAN_POINT('Ctrl Pts',(0.00149999999999995,-0.0234384855154046,
0.0145730058670131));
#29305=CARTESIAN_POINT('Ctrl Pts',(0.00146230406011329,-0.0236394436977337,
0.0145770395249264));
#29306=CARTESIAN_POINT('Ctrl Pts',(0.00130918262072881,-0.0240089732900866,
0.0145915885123658));
#29307=CARTESIAN_POINT('Ctrl Pts',(0.00119376432903963,-0.02417755601452,
0.0146018915486846));
#29308=CARTESIAN_POINT('Ctrl Pts',(0.000927556512672219,-0.0244437638308874,
0.0146212157105804));
#29309=CARTESIAN_POINT('Ctrl Pts',(0.000758973570028422,-0.0245591825115081,
0.0146314951324581));
#29310=CARTESIAN_POINT('Ctrl Pts',(0.00038944324592254,-0.0247123042405513,
0.0146459900535485));
#29311=CARTESIAN_POINT('Ctrl Pts',(0.000188484809983388,-0.02475,0.0146499999999999));
#29312=CARTESIAN_POINT('Ctrl Pts',(-0.000188484809983486,-0.02475,0.0146499999999999));
#29313=CARTESIAN_POINT('Ctrl Pts',(-0.000389443245922638,-0.0247123042405513,
0.0146459900535485));
#29314=CARTESIAN_POINT('Ctrl Pts',(-0.000758973570028519,-0.0245591825115081,
0.0146314951324581));
#29315=CARTESIAN_POINT('Ctrl Pts',(-0.000927556512672316,-0.0244437638308874,
0.0146212157105804));
#29316=CARTESIAN_POINT('Ctrl Pts',(-0.00119376432903973,-0.02417755601452,
0.0146018915486846));
#29317=CARTESIAN_POINT('Ctrl Pts',(-0.0013091826207289,-0.0240089732900866,
0.0145915885123658));
#29318=CARTESIAN_POINT('Ctrl Pts',(-0.00146230406011339,-0.0236394436977337,
0.0145770395249264));
#29319=CARTESIAN_POINT('Ctrl Pts',(-0.00150000000000005,-0.0234384855154046,
0.0145730058670131));
#29320=CARTESIAN_POINT('Ctrl Pts',(-0.00150000000000005,-0.02325,0.0145730058670131));
#29321=CARTESIAN_POINT('Origin',(-0.00463991534334946,-0.00365,0.0131027167261812));
#29322=CARTESIAN_POINT('',(-0.00463991534334946,-0.02475,0.0131027167261812));
#29323=CARTESIAN_POINT('',(-0.00231995767168476,-0.02475000000001,0.00655135836310057));
#29324=CARTESIAN_POINT('',(-0.00463991534334946,-0.00815,0.0131027167261812));
#29325=CARTESIAN_POINT('',(-0.00231995767168476,-0.00814999999999,0.00655135836310057));
#29326=CARTESIAN_POINT('',(-0.00463991534335946,-0.00364999999999,0.0131027167261912));
#29327=CARTESIAN_POINT('Origin',(-0.000905995435036485,-0.0059,0.00705206865194123));
#29328=CARTESIAN_POINT('',(-0.00170263522945404,-0.00365,0.0137953265012257));
#29329=CARTESIAN_POINT('',(0.000507966801611784,-0.00364999999999,0.00755277894080188));
#29330=CARTESIAN_POINT('Origin',(-4.56515315114362E-17,-0.00814999999999,
-6.77116287837691E-17));
#29331=CARTESIAN_POINT('Origin',(-4.56515315114362E-17,-0.00365,-6.77116287837691E-17));
#29332=CARTESIAN_POINT('',(0.00170263522945395,-0.00365,0.0137953265012257));
#29333=CARTESIAN_POINT('',(-0.000382789229399208,-0.00364999999999,0.00790626949996145));
#29334=CARTESIAN_POINT('Origin',(-4.56515315114362E-17,-0.00364999999999,
-6.77116287837691E-17));
#29335=CARTESIAN_POINT('Origin',(0.00103117300724906,-0.0059,0.0074055592111008));
#29336=CARTESIAN_POINT('',(0.00463991534334937,-0.00815,0.0131027167261812));
#29337=CARTESIAN_POINT('Origin',(-4.56515315114362E-17,-0.00814999999999,
-6.77116287837691E-17));
#29338=CARTESIAN_POINT('',(0.00244513524389734,-0.00814999999999,0.00690484892226014));
#29339=CARTESIAN_POINT('Origin',(0.0048902704877747,-0.00365,0.0138096978445003));
#29340=CARTESIAN_POINT('',(0.00463991534334937,-0.02475,0.0131027167261812));
#29341=CARTESIAN_POINT('',(0.00244513524389733,-0.02475000000001,0.00690484892226014));
#29342=CARTESIAN_POINT('',(0.00463991534335937,-0.00364999999999,0.0131027167261912));
#29343=CARTESIAN_POINT('Origin',(0.00103117300724906,-0.027,0.0074055592111008));
#29344=CARTESIAN_POINT('',(0.00170263522945395,-0.02925,0.0137953265012257));
#29345=CARTESIAN_POINT('',(-0.000382789229399207,-0.02925000000001,0.00790626949996145));
#29346=CARTESIAN_POINT('Origin',(-4.56515315114362E-17,-0.02475000000001,
-6.77116287837691E-17));
#29347=CARTESIAN_POINT('Origin',(-4.56515315114362E-17,-0.00365,-6.77116287837691E-17));
#29348=CARTESIAN_POINT('',(-0.00170263522945404,-0.02925,0.0137953265012257));
#29349=CARTESIAN_POINT('Origin',(-4.56515315114362E-17,-0.02475000000001,
-6.77116287837691E-17));
#29350=CARTESIAN_POINT('Origin',(-4.56515315114362E-17,-0.02925000000001,
-6.77116287837691E-17));
#29351=CARTESIAN_POINT('Origin',(-4.56515315114362E-17,-0.02925,-6.77116287837691E-17));
#29352=CARTESIAN_POINT('',(0.000507966801611784,-0.02925000000001,0.00755277894080188));
#29353=CARTESIAN_POINT('Origin',(-0.000905995435036485,-0.027,0.00705206865194123));
#29354=CARTESIAN_POINT('Origin',(0.00149999999999995,-0.00965,0.0184));
#29355=CARTESIAN_POINT('',(0.00149999999999995,-0.00965,0.0184));
#29356=CARTESIAN_POINT('',(0.00150000000000994,-0.00964999999999,0.01840000000001));
#29357=CARTESIAN_POINT('',(0.00149999999999995,-0.02325,0.0184));
#29358=CARTESIAN_POINT('',(0.00150000000000994,-0.00964999999999,0.01840000000001));
#29359=CARTESIAN_POINT('',(0.00150000000000994,-0.02325000000001,0.01840000000001));
#29360=CARTESIAN_POINT('Origin',(-4.89822005853117E-17,-0.00965,0.0184));
#29361=CARTESIAN_POINT('',(-0.00150000000000005,-0.00965,0.0184));
#29362=CARTESIAN_POINT('',(-0.00150000000001004,-0.00964999999999,0.01840000000001));
#29363=CARTESIAN_POINT('Origin',(-1.00489822005853E-14,-0.00964999999999,
0.01840000000001));
#29364=CARTESIAN_POINT('Origin',(-4.89822005853117E-17,-0.02325,0.0184));
#29365=CARTESIAN_POINT('',(-0.00150000000000005,-0.02325,0.0184));
#29366=CARTESIAN_POINT('Origin',(-1.00489822005853E-14,-0.02325000000001,
0.01840000000001));
#29367=CARTESIAN_POINT('',(-0.00150000000001006,-0.02325000000001,0.01840000000001));
#29368=CARTESIAN_POINT('Origin',(-0.00150000000000005,-0.02325,0.0184));
#29369=CARTESIAN_POINT('',(-0.00150000000001004,-0.02325000000001,0.01840000000001));
#29370=CARTESIAN_POINT('Origin',(-4.56515315114362E-17,-0.00365,-6.77116287837691E-17));
#29371=CARTESIAN_POINT('',(0.00888108833605071,-0.02925,0.0116511274118542));
#29372=CARTESIAN_POINT('',(0.00630698756824148,-0.02475,0.0132228744157254));
#29373=CARTESIAN_POINT('Origin',(-4.56515315114362E-17,-0.02475000000001,
-6.77116287837691E-17));
#29374=CARTESIAN_POINT('',(0.0116511274118543,-0.02925,0.00888108833605068));
#29375=CARTESIAN_POINT('Origin',(-4.56515315114362E-17,-0.02925000000001,
-6.77116287837691E-17));
#29376=CARTESIAN_POINT('',(0.0132228744157255,-0.02475,0.00630698756824146));
#29377=CARTESIAN_POINT('Origin',(-4.56515315114362E-17,-0.02475000000001,
-6.77116287837691E-17));
#29378=CARTESIAN_POINT('',(0.0132228744157255,-0.00815,0.00630698756824146));
#29379=CARTESIAN_POINT('',(0.0132228744157355,-0.00364999999999,0.00630698756825146));
#29380=CARTESIAN_POINT('',(0.0116511274118543,-0.00365,0.00888108833605069));
#29381=CARTESIAN_POINT('Origin',(-4.56515315114362E-17,-0.00814999999999,
-6.77116287837691E-17));
#29382=CARTESIAN_POINT('',(0.00888108833605071,-0.00365,0.0116511274118542));
#29383=CARTESIAN_POINT('Origin',(-4.56515315114362E-17,-0.00364999999999,
-6.77116287837691E-17));
#29384=CARTESIAN_POINT('',(0.00630698756824148,-0.00815,0.0132228744157254));
#29385=CARTESIAN_POINT('Origin',(-4.56515315114362E-17,-0.00814999999999,
-6.77116287837691E-17));
#29386=CARTESIAN_POINT('',(0.00630698756825148,-0.00364999999999,0.0132228744157354));
#29387=CARTESIAN_POINT('',(0.00924401109905649,-0.02325,0.0113653314426161));
#29388=CARTESIAN_POINT('',(0.00924401109905649,-0.00965,0.0113653314426161));
#29389=CARTESIAN_POINT('',(0.00924401109906649,-0.00364999999999,0.0113653314426261));
#29390=CARTESIAN_POINT('',(0.0113653314426162,-0.00965,0.00924401109905646));
#29391=CARTESIAN_POINT('Ctrl Pts',(0.00924401109905653,-0.00965,0.0113653314426161));
#29392=CARTESIAN_POINT('Ctrl Pts',(0.00924401109905653,-0.00946151448459537,
0.0113653314426161));
#29393=CARTESIAN_POINT('Ctrl Pts',(0.00927351838063707,-0.00926055630226629,
0.0113415286147625));
#29394=CARTESIAN_POINT('Ctrl Pts',(0.00939207927644866,-0.00889102670991339,
0.0112435430943065));
#29395=CARTESIAN_POINT('Ctrl Pts',(0.00948097768002293,-0.00872244398548004,
0.011169215384428));
#29396=CARTESIAN_POINT('Ctrl Pts',(0.00968287927809845,-0.00845623616911263,
0.010994642278187));
#29397=CARTESIAN_POINT('Ctrl Pts',(0.00980935406895063,-0.00834081748849188,
0.0108827047851675));
#29398=CARTESIAN_POINT('Ctrl Pts',(0.0100809009239757,-0.00818769575944872,
0.0106316568441339));
#29399=CARTESIAN_POINT('Ctrl Pts',(0.010225835457093,-0.00815,0.0104923932316728));
#29400=CARTESIAN_POINT('Ctrl Pts',(0.0104923932316729,-0.00815,0.0102258354570929));
#29401=CARTESIAN_POINT('Ctrl Pts',(0.0106316568441341,-0.00818769575944871,
0.0100809009239756));
#29402=CARTESIAN_POINT('Ctrl Pts',(0.0108827047851676,-0.00834081748849188,
0.00980935406895052));
#29403=CARTESIAN_POINT('Ctrl Pts',(0.0109946422781871,-0.00845623616911263,
0.00968287927809834));
#29404=CARTESIAN_POINT('Ctrl Pts',(0.0111692153844281,-0.00872244398548004,
0.00948097768002282));
#29405=CARTESIAN_POINT('Ctrl Pts',(0.0112435430943066,-0.00889102670991339,
0.00939207927644855));
#29406=CARTESIAN_POINT('Ctrl Pts',(0.0113415286147626,-0.00926055630226629,
0.00927351838063695));
#29407=CARTESIAN_POINT('Ctrl Pts',(0.0113653314426162,-0.00946151448459537,
0.00924401109905641));
#29408=CARTESIAN_POINT('Ctrl Pts',(0.0113653314426162,-0.00965,0.00924401109905641));
#29409=CARTESIAN_POINT('',(0.0113653314426162,-0.02325,0.00924401109905646));
#29410=CARTESIAN_POINT('',(0.0113653314426262,-0.00364999999999,0.00924401109906647));
#29411=CARTESIAN_POINT('Ctrl Pts',(0.0113653314426162,-0.02325,0.00924401109905641));
#29412=CARTESIAN_POINT('Ctrl Pts',(0.0113653314426162,-0.0234384855154046,
0.00924401109905641));
#29413=CARTESIAN_POINT('Ctrl Pts',(0.0113415286147626,-0.0236394436977337,
0.00927351838063695));
#29414=CARTESIAN_POINT('Ctrl Pts',(0.0112435430943066,-0.0240089732900866,
0.00939207927644855));
#29415=CARTESIAN_POINT('Ctrl Pts',(0.0111692153844281,-0.02417755601452,
0.00948097768002282));
#29416=CARTESIAN_POINT('Ctrl Pts',(0.0109946422781871,-0.0244437638308874,
0.00968287927809834));
#29417=CARTESIAN_POINT('Ctrl Pts',(0.0108827047851676,-0.0245591825115081,
0.00980935406895052));
#29418=CARTESIAN_POINT('Ctrl Pts',(0.0106316568441341,-0.0247123042405513,
0.0100809009239756));
#29419=CARTESIAN_POINT('Ctrl Pts',(0.0104923932316729,-0.02475,0.0102258354570929));
#29420=CARTESIAN_POINT('Ctrl Pts',(0.010225835457093,-0.02475,0.0104923932316728));
#29421=CARTESIAN_POINT('Ctrl Pts',(0.0100809009239757,-0.0247123042405513,
0.0106316568441339));
#29422=CARTESIAN_POINT('Ctrl Pts',(0.00980935406895063,-0.0245591825115081,
0.0108827047851675));
#29423=CARTESIAN_POINT('Ctrl Pts',(0.00968287927809845,-0.0244437638308874,
0.010994642278187));
#29424=CARTESIAN_POINT('Ctrl Pts',(0.00948097768002293,-0.02417755601452,
0.011169215384428));
#29425=CARTESIAN_POINT('Ctrl Pts',(0.00939207927644866,-0.0240089732900866,
0.0112435430943065));
#29426=CARTESIAN_POINT('Ctrl Pts',(0.00927351838063707,-0.0236394436977337,
0.0113415286147625));
#29427=CARTESIAN_POINT('Ctrl Pts',(0.00924401109905653,-0.0234384855154046,
0.0113653314426161));
#29428=CARTESIAN_POINT('Ctrl Pts',(0.00924401109905653,-0.02325,0.0113653314426161));
#29429=CARTESIAN_POINT('Origin',(0.00598410424563526,-0.00365,0.012545935452463));
#29430=CARTESIAN_POINT('',(0.00598410424563526,-0.02475,0.012545935452463));
#29431=CARTESIAN_POINT('',(0.00299205212282761,-0.02475000000001,0.00627296772624146));
#29432=CARTESIAN_POINT('',(0.00598410424563526,-0.00815,0.012545935452463));
#29433=CARTESIAN_POINT('',(0.00299205212282761,-0.00814999999999,0.00627296772624146));
#29434=CARTESIAN_POINT('',(0.00598410424564526,-0.00364999999999,0.012545935452473));
#29435=CARTESIAN_POINT('Origin',(0.0043459300493424,-0.0059,0.00562720108101902));
#29436=CARTESIAN_POINT('',(0.00855082400106517,-0.00365,0.0109587138343332));
#29437=CARTESIAN_POINT('',(0.00569980797587718,-0.00364999999999,0.00498143443581658));
#29438=CARTESIAN_POINT('Origin',(-4.56515315114362E-17,-0.00814999999999,
-6.77116287837691E-17));
#29439=CARTESIAN_POINT('Origin',(-4.56515315114362E-17,-0.00365,-6.77116287837691E-17));
#29440=CARTESIAN_POINT('',(0.0109587138343332,-0.00365,0.00855082400106514));
#29441=CARTESIAN_POINT('',(0.0053199039174478,-0.00364999999999,0.00586124963718028));
#29442=CARTESIAN_POINT('Origin',(-4.56515315114362E-17,-0.00364999999999,
-6.77116287837691E-17));
#29443=CARTESIAN_POINT('Origin',(0.00596567056265024,-0.0059,0.00450737171064548));
#29444=CARTESIAN_POINT('',(0.0125459354524631,-0.00815,0.00598410424563523));
#29445=CARTESIAN_POINT('Origin',(-4.56515315114362E-17,-0.00814999999999,
-6.77116287837691E-17));
#29446=CARTESIAN_POINT('',(0.00661143720787268,-0.00814999999999,0.0031534937841307));
#29447=CARTESIAN_POINT('Origin',(0.0132228744157255,-0.00365,0.00630698756824145));
#29448=CARTESIAN_POINT('',(0.0125459354524631,-0.02475,0.00598410424563523));
#29449=CARTESIAN_POINT('',(0.00661143720787268,-0.02475000000001,0.0031534937841307));
#29450=CARTESIAN_POINT('',(0.0125459354524731,-0.00364999999999,0.00598410424564523));
#29451=CARTESIAN_POINT('Origin',(0.00596567056265024,-0.027,0.00450737171064548));
#29452=CARTESIAN_POINT('',(0.0109587138343332,-0.02925,0.00855082400106514));
#29453=CARTESIAN_POINT('',(0.0053199039174478,-0.02925000000001,0.00586124963718027));
#29454=CARTESIAN_POINT('Origin',(-4.56515315114362E-17,-0.02475000000001,
-6.77116287837691E-17));
#29455=CARTESIAN_POINT('Origin',(-4.56515315114362E-17,-0.00365,-6.77116287837691E-17));
#29456=CARTESIAN_POINT('',(0.00855082400106517,-0.02925,0.0109587138343332));
#29457=CARTESIAN_POINT('Origin',(-4.56515315114362E-17,-0.02475000000001,
-6.77116287837691E-17));
#29458=CARTESIAN_POINT('Origin',(-4.56515315114362E-17,-0.02925000000001,
-6.77116287837691E-17));
#29459=CARTESIAN_POINT('Origin',(-4.56515315114362E-17,-0.02925,-6.77116287837691E-17));
#29460=CARTESIAN_POINT('',(0.00569980797587718,-0.02925000000001,0.00498143443581658));
#29461=CARTESIAN_POINT('Origin',(0.0043459300493424,-0.027,0.00562720108101902));
#29462=CARTESIAN_POINT('Origin',(0.0140714249456123,-0.00965,0.0119501046020526));
#29463=CARTESIAN_POINT('',(0.0140714249456123,-0.00965,0.0119501046020526));
#29464=CARTESIAN_POINT('',(0.0140714249456223,-0.00964999999999,0.0119501046020626));
#29465=CARTESIAN_POINT('',(0.0140714249456123,-0.02325,0.0119501046020526));
#29466=CARTESIAN_POINT('',(0.0140714249456223,-0.00964999999999,0.0119501046020626));
#29467=CARTESIAN_POINT('',(0.0140714249456223,-0.02325000000001,0.0119501046020626));
#29468=CARTESIAN_POINT('Origin',(0.0130107647738325,-0.00965,0.0130107647738324));
#29469=CARTESIAN_POINT('',(0.0119501046020527,-0.00965,0.0140714249456122));
#29470=CARTESIAN_POINT('',(0.0119501046020627,-0.00964999999999,0.0140714249456222));
#29471=CARTESIAN_POINT('Origin',(0.0130107647738425,-0.00964999999999,0.0130107647738424));
#29472=CARTESIAN_POINT('Origin',(0.0130107647738325,-0.02325,0.0130107647738324));
#29473=CARTESIAN_POINT('',(0.0119501046020527,-0.02325,0.0140714249456122));
#29474=CARTESIAN_POINT('Origin',(0.0130107647738425,-0.02325000000001,0.0130107647738424));
#29475=CARTESIAN_POINT('',(0.0119501046020627,-0.02325000000001,0.0140714249456222));
#29476=CARTESIAN_POINT('Origin',(0.0119501046020527,-0.02325,0.0140714249456122));
#29477=CARTESIAN_POINT('',(0.0119501046020627,-0.02325000000001,0.0140714249456222));
#29478=CARTESIAN_POINT('Origin',(-4.56515315114362E-17,-0.00365,-6.77116287837691E-17));
#29479=CARTESIAN_POINT('',(0.0145184689881289,-0.02925,0.00195871341465235));
#29480=CARTESIAN_POINT('',(0.0138096978445004,-0.02475,0.00489027048777468));
#29481=CARTESIAN_POINT('Origin',(-4.56515315114362E-17,-0.02475000000001,
-6.77116287837691E-17));
#29482=CARTESIAN_POINT('',(0.0145184689881289,-0.02925,-0.00195871341465249));
#29483=CARTESIAN_POINT('Origin',(-4.56515315114362E-17,-0.02925000000001,
-6.77116287837691E-17));
#29484=CARTESIAN_POINT('',(0.0138096978445004,-0.02475,-0.00489027048777481));
#29485=CARTESIAN_POINT('Origin',(-4.56515315114362E-17,-0.02475000000001,
-6.77116287837691E-17));
#29486=CARTESIAN_POINT('',(0.0138096978445004,-0.00815,-0.00489027048777481));
#29487=CARTESIAN_POINT('',(0.0138096978445104,-0.00364999999999,-0.00489027048778481));
#29488=CARTESIAN_POINT('',(0.0145184689881289,-0.00365,-0.00195871341465249));
#29489=CARTESIAN_POINT('Origin',(-4.56515315114362E-17,-0.00814999999999,
-6.77116287837691E-17));
#29490=CARTESIAN_POINT('',(0.0145184689881289,-0.00365,0.00195871341465235));
#29491=CARTESIAN_POINT('Origin',(-4.56515315114362E-17,-0.00364999999999,
-6.77116287837691E-17));
#29492=CARTESIAN_POINT('',(0.0138096978445004,-0.00815,0.00489027048777468));
#29493=CARTESIAN_POINT('Origin',(-4.56515315114362E-17,-0.00814999999999,
-6.77116287837691E-17));
#29494=CARTESIAN_POINT('',(0.0138096978445104,-0.00364999999999,0.00489027048778468));
#29495=CARTESIAN_POINT('',(0.0145730058670132,-0.02325,0.00149999999999993));
#29496=CARTESIAN_POINT('',(0.0145730058670132,-0.00965,0.00149999999999993));
#29497=CARTESIAN_POINT('',(0.0145730058670232,-0.00364999999999,0.00150000000000994));
#29498=CARTESIAN_POINT('',(0.0145730058670132,-0.00965,-0.00150000000000007));
#29499=CARTESIAN_POINT('Ctrl Pts',(0.0145730058670131,-0.00965,0.00149999999999993));
#29500=CARTESIAN_POINT('Ctrl Pts',(0.0145730058670131,-0.00946151448459537,
0.00149999999999993));
#29501=CARTESIAN_POINT('Ctrl Pts',(0.0145770395249264,-0.00926055630226629,
0.00146230406011328));
#29502=CARTESIAN_POINT('Ctrl Pts',(0.0145915885123658,-0.00889102670991339,
0.00130918262072879));
#29503=CARTESIAN_POINT('Ctrl Pts',(0.0146018915486847,-0.00872244398548004,
0.00119376432903961));
#29504=CARTESIAN_POINT('Ctrl Pts',(0.0146212157105804,-0.00845623616911263,
0.000927556512672201));
#29505=CARTESIAN_POINT('Ctrl Pts',(0.0146314951324581,-0.00834081748849188,
0.000758973570028406));
#29506=CARTESIAN_POINT('Ctrl Pts',(0.0146459900535485,-0.00818769575944871,
0.000389443245922524));
#29507=CARTESIAN_POINT('Ctrl Pts',(0.01465,-0.00815,0.000188484809983372));
#29508=CARTESIAN_POINT('Ctrl Pts',(0.01465,-0.00815,-0.000188484809983502));
#29509=CARTESIAN_POINT('Ctrl Pts',(0.0146459900535485,-0.00818769575944871,
-0.000389443245922654));
#29510=CARTESIAN_POINT('Ctrl Pts',(0.0146314951324581,-0.00834081748849188,
-0.000758973570028536));
#29511=CARTESIAN_POINT('Ctrl Pts',(0.0146212157105804,-0.00845623616911263,
-0.000927556512672332));
#29512=CARTESIAN_POINT('Ctrl Pts',(0.0146018915486847,-0.00872244398548004,
-0.00119376432903974));
#29513=CARTESIAN_POINT('Ctrl Pts',(0.0145915885123658,-0.00889102670991339,
-0.00130918262072892));
#29514=CARTESIAN_POINT('Ctrl Pts',(0.0145770395249264,-0.00926055630226629,
-0.00146230406011341));
#29515=CARTESIAN_POINT('Ctrl Pts',(0.0145730058670131,-0.00946151448459537,
-0.00150000000000006));
#29516=CARTESIAN_POINT('Ctrl Pts',(0.0145730058670131,-0.00965,-0.00150000000000006));
#29517=CARTESIAN_POINT('',(0.0145730058670132,-0.02325,-0.00150000000000007));
#29518=CARTESIAN_POINT('',(0.0145730058670232,-0.00364999999999,-0.00150000000001006));
#29519=CARTESIAN_POINT('Ctrl Pts',(0.0145730058670131,-0.02325,-0.00150000000000007));
#29520=CARTESIAN_POINT('Ctrl Pts',(0.0145730058670131,-0.0234384855154046,
-0.00150000000000007));
#29521=CARTESIAN_POINT('Ctrl Pts',(0.0145770395249264,-0.0236394436977337,
-0.00146230406011341));
#29522=CARTESIAN_POINT('Ctrl Pts',(0.0145915885123658,-0.0240089732900866,
-0.00130918262072892));
#29523=CARTESIAN_POINT('Ctrl Pts',(0.0146018915486847,-0.02417755601452,
-0.00119376432903974));
#29524=CARTESIAN_POINT('Ctrl Pts',(0.0146212157105804,-0.0244437638308874,
-0.000927556512672333));
#29525=CARTESIAN_POINT('Ctrl Pts',(0.0146314951324581,-0.0245591825115081,
-0.000758973570028536));
#29526=CARTESIAN_POINT('Ctrl Pts',(0.0146459900535485,-0.0247123042405513,
-0.000389443245922655));
#29527=CARTESIAN_POINT('Ctrl Pts',(0.01465,-0.02475,-0.000188484809983502));
#29528=CARTESIAN_POINT('Ctrl Pts',(0.0146499999999999,-0.02475,0.000188484809983372));
#29529=CARTESIAN_POINT('Ctrl Pts',(0.0146459900535485,-0.0247123042405513,
0.000389443245922527));
#29530=CARTESIAN_POINT('Ctrl Pts',(0.0146314951324581,-0.0245591825115081,
0.000758973570028408));
#29531=CARTESIAN_POINT('Ctrl Pts',(0.0146212157105804,-0.0244437638308874,
0.000927556512672202));
#29532=CARTESIAN_POINT('Ctrl Pts',(0.0146018915486847,-0.02417755601452,
0.00119376432903961));
#29533=CARTESIAN_POINT('Ctrl Pts',(0.0145915885123658,-0.0240089732900866,
0.00130918262072879));
#29534=CARTESIAN_POINT('Ctrl Pts',(0.0145770395249264,-0.0236394436977337,
0.00146230406011327));
#29535=CARTESIAN_POINT('Ctrl Pts',(0.0145730058670131,-0.0234384855154046,
0.00149999999999993));
#29536=CARTESIAN_POINT('Ctrl Pts',(0.0145730058670131,-0.02325,0.00149999999999993));
#29537=CARTESIAN_POINT('Origin',(0.0131027167261813,-0.00365,0.00463991534334935));
#29538=CARTESIAN_POINT('',(0.0131027167261813,-0.02475,0.00463991534334935));
#29539=CARTESIAN_POINT('',(0.00655135836310059,-0.02475000000001,0.00231995767168465));
#29540=CARTESIAN_POINT('',(0.0131027167261813,-0.00815,0.00463991534334935));
#29541=CARTESIAN_POINT('',(0.00655135836310059,-0.00814999999999,0.00231995767168465));
#29542=CARTESIAN_POINT('',(0.0131027167261912,-0.00364999999999,0.00463991534335935));
#29543=CARTESIAN_POINT('Origin',(0.00705206865194125,-0.0059,0.000905995435036372));
#29544=CARTESIAN_POINT('',(0.0137953265012258,-0.00365,0.00170263522945392));
#29545=CARTESIAN_POINT('',(0.0075527789408019,-0.00364999999999,-0.000507966801611896));
#29546=CARTESIAN_POINT('Origin',(-4.56515315114362E-17,-0.00814999999999,
-6.77116287837691E-17));
#29547=CARTESIAN_POINT('Origin',(-4.56515315114362E-17,-0.00365,-6.77116287837691E-17));
#29548=CARTESIAN_POINT('',(0.0137953265012258,-0.00365,-0.00170263522945406));
#29549=CARTESIAN_POINT('',(0.00790626949996147,-0.00364999999999,0.000382789229399096));
#29550=CARTESIAN_POINT('Origin',(-4.56515315114362E-17,-0.00364999999999,
-6.77116287837691E-17));
#29551=CARTESIAN_POINT('Origin',(0.00740555921110082,-0.0059,-0.00103117300724917));
#29552=CARTESIAN_POINT('',(0.0131027167261813,-0.00815,-0.00463991534334949));
#29553=CARTESIAN_POINT('Origin',(-4.56515315114362E-17,-0.00814999999999,
-6.77116287837691E-17));
#29554=CARTESIAN_POINT('',(0.00690484892226016,-0.00814999999999,-0.00244513524389744));
#29555=CARTESIAN_POINT('Origin',(0.0138096978445004,-0.00365,-0.00489027048777482));
#29556=CARTESIAN_POINT('',(0.0131027167261813,-0.02475,-0.00463991534334949));
#29557=CARTESIAN_POINT('',(0.00690484892226016,-0.02475000000001,-0.00244513524389744));
#29558=CARTESIAN_POINT('',(0.0131027167261912,-0.00364999999999,-0.00463991534335949));
#29559=CARTESIAN_POINT('Origin',(0.00740555921110082,-0.027,-0.00103117300724918));
#29560=CARTESIAN_POINT('',(0.0137953265012258,-0.02925,-0.00170263522945406));
#29561=CARTESIAN_POINT('',(0.00790626949996147,-0.02925000000001,0.000382789229399094));
#29562=CARTESIAN_POINT('Origin',(-4.56515315114362E-17,-0.02475000000001,
-6.77116287837691E-17));
#29563=CARTESIAN_POINT('Origin',(-4.56515315114362E-17,-0.00365,-6.77116287837691E-17));
#29564=CARTESIAN_POINT('',(0.0137953265012258,-0.02925,0.00170263522945392));
#29565=CARTESIAN_POINT('Origin',(-4.56515315114362E-17,-0.02475000000001,
-6.77116287837691E-17));
#29566=CARTESIAN_POINT('Origin',(-4.56515315114362E-17,-0.02925000000001,
-6.77116287837691E-17));
#29567=CARTESIAN_POINT('Origin',(-4.56515315114362E-17,-0.02925,-6.77116287837691E-17));
#29568=CARTESIAN_POINT('',(0.0075527789408019,-0.02925000000001,-0.000507966801611896));
#29569=CARTESIAN_POINT('Origin',(0.00705206865194125,-0.027,0.000905995435036372));
#29570=CARTESIAN_POINT('Origin',(0.0184,-0.00965,-0.00150000000000007));
#29571=CARTESIAN_POINT('',(0.0184,-0.00965,-0.00150000000000007));
#29572=CARTESIAN_POINT('',(0.01840000000001,-0.00964999999999,-0.00150000000001006));
#29573=CARTESIAN_POINT('',(0.0184,-0.02325,-0.00150000000000007));
#29574=CARTESIAN_POINT('',(0.01840000000001,-0.00964999999999,-0.00150000000001006));
#29575=CARTESIAN_POINT('',(0.01840000000001,-0.02325000000001,-0.00150000000001006));
#29576=CARTESIAN_POINT('Origin',(0.0184,-0.00965,-6.43809597098936E-17));
#29577=CARTESIAN_POINT('',(0.0184,-0.00965,0.00149999999999993));
#29578=CARTESIAN_POINT('',(0.01840000000001,-0.00964999999999,0.00150000000000994));
#29579=CARTESIAN_POINT('Origin',(0.01840000000001,-0.00964999999999,9.93561904029011E-15));
#29580=CARTESIAN_POINT('Origin',(0.0184,-0.02325,-6.43809597098936E-17));
#29581=CARTESIAN_POINT('',(0.0184,-0.024,-0.00129903810567673));
#29582=CARTESIAN_POINT('Origin',(0.01840000000001,-0.02325000000001,9.93561904029011E-15));
#29583=CARTESIAN_POINT('',(0.0184,-0.024,0.00129903810567659));
#29584=CARTESIAN_POINT('Origin',(0.01840000000001,-0.02325000000001,9.93561904029011E-15));
#29585=CARTESIAN_POINT('',(0.0184,-0.02325,0.00149999999999993));
#29586=CARTESIAN_POINT('Origin',(0.01840000000001,-0.02325000000001,9.93561904029011E-15));
#29587=CARTESIAN_POINT('',(0.01840000000001,-0.02325000000001,0.00150000000000994));
#29588=CARTESIAN_POINT('Origin',(0.0184,-0.02325,0.00149999999999993));
#29589=CARTESIAN_POINT('',(0.01840000000001,-0.02325000000001,0.00150000000000994));
#29590=CARTESIAN_POINT('Origin',(-4.78719775606865E-17,-0.00365,-6.88218518083943E-17));
#29591=CARTESIAN_POINT('',(0.01915,-0.00365,0.00793218971944471));
#29592=CARTESIAN_POINT('',(0.01915,-0.00365,-0.00793218971944484));
#29593=CARTESIAN_POINT('',(0.01915000000001,-0.00364999999999,0.00793218971945471));
#29594=CARTESIAN_POINT('',(0.00793218971944474,-0.00365,-0.01915));
#29595=CARTESIAN_POINT('',(0.01915000000001,-0.00364999999999,-0.00793218971945484));
#29596=CARTESIAN_POINT('',(-0.00793218971944482,-0.00365,-0.01915));
#29597=CARTESIAN_POINT('',(0.00793218971945473,-0.00364999999999,-0.0191500000000101));
#29598=CARTESIAN_POINT('',(-0.01915,-0.00365,-0.00793218971944485));
#29599=CARTESIAN_POINT('',(-0.00793218971945482,-0.00364999999999,-0.0191500000000101));
#29600=CARTESIAN_POINT('',(-0.01915,-0.00365,0.0079321897194447));
#29601=CARTESIAN_POINT('',(-0.0191500000000101,-0.00364999999999,-0.00793218971945485));
#29602=CARTESIAN_POINT('',(-0.00793218971944483,-0.00365,0.01915));
#29603=CARTESIAN_POINT('',(-0.0191500000000101,-0.00364999999999,0.0079321897194547));
#29604=CARTESIAN_POINT('',(0.00793218971944473,-0.00365,0.01915));
#29605=CARTESIAN_POINT('',(-0.00793218971945483,-0.00364999999999,0.01915000000001));
#29606=CARTESIAN_POINT('',(0.00793218971945473,-0.00364999999999,0.01915000000001));
#29607=CARTESIAN_POINT('',(0.0184,-0.00365,-0.00762152954766502));
#29608=CARTESIAN_POINT('',(0.0184,-0.00365,0.00762152954766488));
#29609=CARTESIAN_POINT('',(0.01840000000001,-0.00364999999999,-0.00762152954767502));
#29610=CARTESIAN_POINT('',(0.0076215295476649,-0.00365,0.0184));
#29611=CARTESIAN_POINT('',(0.01840000000001,-0.00364999999999,0.00762152954767488));
#29612=CARTESIAN_POINT('',(-0.007621529547665,-0.00365,0.0184));
#29613=CARTESIAN_POINT('',(0.0076215295476749,-0.00364999999999,0.01840000000001));
#29614=CARTESIAN_POINT('',(-0.0184,-0.00365,0.00762152954766489));
#29615=CARTESIAN_POINT('',(-0.007621529547675,-0.00364999999999,0.01840000000001));
#29616=CARTESIAN_POINT('',(-0.0184,-0.00365,-0.00762152954766502));
#29617=CARTESIAN_POINT('',(-0.0184000000000101,-0.00364999999999,0.00762152954767489));
#29618=CARTESIAN_POINT('',(-0.007621529547665,-0.00365,-0.0184));
#29619=CARTESIAN_POINT('',(-0.0184000000000101,-0.00364999999999,-0.00762152954767502));
#29620=CARTESIAN_POINT('',(0.00762152954766491,-0.00365,-0.0184));
#29621=CARTESIAN_POINT('',(-0.007621529547675,-0.00364999999999,-0.0184000000000101));
#29622=CARTESIAN_POINT('',(0.00762152954767491,-0.00364999999999,-0.0184000000000101));
#29623=CARTESIAN_POINT('Origin',(-0.01915,-0.01645,0.0079321897194447));
#29624=CARTESIAN_POINT('',(-0.00793218971944483,-0.02925,0.01915));
#29625=CARTESIAN_POINT('',(-0.00793218971945483,-0.01645,0.01915000000001));
#29626=CARTESIAN_POINT('',(-0.01915,-0.02925,0.0079321897194447));
#29627=CARTESIAN_POINT('',(-0.0191500000000101,-0.01645,0.0079321897194547));
#29628=CARTESIAN_POINT('',(-0.0191500000000101,-0.02925000000001,0.0079321897194547));
#29629=CARTESIAN_POINT('Origin',(-0.00793218971944483,-0.01645,0.01915));
#29630=CARTESIAN_POINT('',(0.00793218971944473,-0.02925,0.01915));
#29631=CARTESIAN_POINT('',(0.00793218971945473,-0.01645,0.01915000000001));
#29632=CARTESIAN_POINT('',(-0.00793218971945483,-0.02925000000001,0.01915000000001));
#29633=CARTESIAN_POINT('Origin',(0.00793218971944473,-0.01645,0.01915));
#29634=CARTESIAN_POINT('',(0.01915,-0.02925,0.00793218971944471));
#29635=CARTESIAN_POINT('',(0.01915,-0.024,0.00793218971944471));
#29636=CARTESIAN_POINT('',(0.01915000000001,-0.01645,0.00793218971945471));
#29637=CARTESIAN_POINT('',(0.01915000000001,-0.01645,0.00793218971945471));
#29638=CARTESIAN_POINT('',(0.00793218971945473,-0.02925000000001,0.01915000000001));
#29639=CARTESIAN_POINT('Origin',(0.01915,-0.01645,-0.00793218971944484));
#29640=CARTESIAN_POINT('',(0.00793218971944474,-0.02925,-0.01915));
#29641=CARTESIAN_POINT('',(0.00793218971945474,-0.01645,-0.0191500000000101));
#29642=CARTESIAN_POINT('',(0.01915,-0.024,-0.00793218971944484));
#29643=CARTESIAN_POINT('',(0.01915000000001,-0.01645,-0.00793218971945484));
#29644=CARTESIAN_POINT('',(0.01915,-0.02925,-0.00793218971944484));
#29645=CARTESIAN_POINT('',(0.01915000000001,-0.01645,-0.00793218971945484));
#29646=CARTESIAN_POINT('',(0.01915000000001,-0.02925000000001,-0.00793218971945484));
#29647=CARTESIAN_POINT('Origin',(0.00793218971944474,-0.01645,-0.01915));
#29648=CARTESIAN_POINT('',(-0.00793218971944482,-0.02925,-0.01915));
#29649=CARTESIAN_POINT('',(-0.00793218971945482,-0.01645,-0.0191500000000101));
#29650=CARTESIAN_POINT('',(0.00793218971945473,-0.02925000000001,-0.0191500000000101));
#29651=CARTESIAN_POINT('Origin',(-0.00793218971944482,-0.01645,-0.01915));
#29652=CARTESIAN_POINT('',(-0.01915,-0.02925,-0.00793218971944485));
#29653=CARTESIAN_POINT('',(-0.0191500000000101,-0.01645,-0.00793218971945485));
#29654=CARTESIAN_POINT('',(-0.00793218971945482,-0.02925000000001,-0.0191500000000101));
#29655=CARTESIAN_POINT('Origin',(-0.01915,-0.01645,-0.00793218971944485));
#29656=CARTESIAN_POINT('',(-0.0191500000000101,-0.02925000000001,-0.00793218971945485));
#29657=CARTESIAN_POINT('Origin',(-4.78719775606865E-17,-0.02925,-6.88218518083943E-17));
#29658=CARTESIAN_POINT('',(0.02715,-0.02925,-0.00793218971944484));
#29659=CARTESIAN_POINT('',(0.01915000000001,-0.02925000000001,-0.00793218971945484));
#29660=CARTESIAN_POINT('',(0.02715,-0.02925,0.00793218971943127));
#29661=CARTESIAN_POINT('',(0.02715000000001,-0.02925000000001,0.00793218971944127));
#29662=CARTESIAN_POINT('',(0.01915000000001,-0.02925000000001,0.00793218971944127));
#29663=CARTESIAN_POINT('',(0.0224,-0.02925,-0.00718218971944484));
#29664=CARTESIAN_POINT('',(0.0184,-0.02925,-0.00718218971944484));
#29665=CARTESIAN_POINT('',(0.01120000000001,-0.02925000000001,-0.00718218971945484));
#29666=CARTESIAN_POINT('',(0.0184,-0.02925,-0.00762152954766502));
#29667=CARTESIAN_POINT('',(0.01840000000001,-0.02925000000001,-0.00762152954767502));
#29668=CARTESIAN_POINT('',(0.00762152954766491,-0.02925,-0.0184));
#29669=CARTESIAN_POINT('',(0.00762152954767491,-0.02925000000001,-0.0184000000000101));
#29670=CARTESIAN_POINT('',(-0.007621529547665,-0.02925,-0.0184));
#29671=CARTESIAN_POINT('',(-0.007621529547675,-0.02925000000001,-0.0184000000000101));
#29672=CARTESIAN_POINT('',(-0.0184,-0.02925,-0.00762152954766502));
#29673=CARTESIAN_POINT('',(-0.0184000000000101,-0.02925000000001,-0.00762152954767502));
#29674=CARTESIAN_POINT('',(-0.0184,-0.02925,0.00762152954766489));
#29675=CARTESIAN_POINT('',(-0.0184000000000101,-0.02925000000001,0.00762152954767489));
#29676=CARTESIAN_POINT('',(-0.007621529547665,-0.02925,0.0184));
#29677=CARTESIAN_POINT('',(-0.007621529547675,-0.02925000000001,0.01840000000001));
#29678=CARTESIAN_POINT('',(0.0076215295476649,-0.02925,0.0184));
#29679=CARTESIAN_POINT('',(0.0076215295476749,-0.02925000000001,0.01840000000001));
#29680=CARTESIAN_POINT('',(0.0184,-0.02925,0.00762152954766488));
#29681=CARTESIAN_POINT('',(0.01840000000001,-0.02925000000001,0.00762152954767488));
#29682=CARTESIAN_POINT('',(0.0184,-0.02925,0.00718218971944471));
#29683=CARTESIAN_POINT('',(0.01840000000001,-0.02925000000001,-0.00762152954767502));
#29684=CARTESIAN_POINT('',(0.0224,-0.02925,0.00718218971944471));
#29685=CARTESIAN_POINT('',(0.00920000000000996,-0.02925000000001,0.00718218971945471));
#29686=CARTESIAN_POINT('',(0.02240000000001,-0.02925000000001,0.00359109485973232));
#29687=CARTESIAN_POINT('Origin',(0.0184,-0.01645,0.00762152954766488));
#29688=CARTESIAN_POINT('',(0.01840000000001,-0.01645,0.00762152954767488));
#29689=CARTESIAN_POINT('',(0.0076215295476749,-0.01645,0.01840000000001));
#29690=CARTESIAN_POINT('Origin',(0.0076215295476649,-0.01645,0.0184));
#29691=CARTESIAN_POINT('',(-0.007621529547675,-0.01645,0.01840000000001));
#29692=CARTESIAN_POINT('Origin',(-0.007621529547665,-0.01645,0.0184));
#29693=CARTESIAN_POINT('',(-0.0184000000000101,-0.01645,0.00762152954767489));
#29694=CARTESIAN_POINT('Origin',(-0.0184,-0.01645,0.00762152954766489));
#29695=CARTESIAN_POINT('',(-0.0184000000000101,-0.01645,-0.00762152954767502));
#29696=CARTESIAN_POINT('Origin',(-0.0184,-0.01645,-0.00762152954766502));
#29697=CARTESIAN_POINT('',(-0.007621529547675,-0.01645,-0.0184000000000101));
#29698=CARTESIAN_POINT('Origin',(-0.007621529547665,-0.01645,-0.0184));
#29699=CARTESIAN_POINT('',(0.00762152954767491,-0.01645,-0.0184000000000101));
#29700=CARTESIAN_POINT('Origin',(0.00762152954766491,-0.01645,-0.0184));
#29701=CARTESIAN_POINT('',(0.01840000000001,-0.01645,-0.00762152954767502));
#29702=CARTESIAN_POINT('Origin',(0.01915,-0.024,0.00718218971944471));
#29703=CARTESIAN_POINT('',(0.0184,-0.024,-0.00718218971944484));
#29704=CARTESIAN_POINT('',(0.01840000000001,-0.02400000000001,-0.000219669914120157));
#29705=CARTESIAN_POINT('',(0.01915,-0.024,-0.00718218971944484));
#29706=CARTESIAN_POINT('',(0.01915000000001,-0.02400000000001,-0.00718218971945484));
#29707=CARTESIAN_POINT('',(0.01915,-0.024,0.00718218971944471));
#29708=CARTESIAN_POINT('',(0.01915000000001,-0.02400000000001,0.00755718971945471));
#29709=CARTESIAN_POINT('',(0.0184,-0.024,0.00718218971944471));
#29710=CARTESIAN_POINT('',(0.01915000000001,-0.02400000000001,0.00718218971945471));
#29711=CARTESIAN_POINT('',(0.01840000000001,-0.02400000000001,-0.000219669914120157));
#29712=CARTESIAN_POINT('',(0.01840000000001,-0.02400000000001,0.00359109485973232));
#29713=CARTESIAN_POINT('Origin',(0.01915,-0.024,-0.00718218971944484));
#29714=CARTESIAN_POINT('',(0.02715,-0.0285,-0.00718218971944484));
#29715=CARTESIAN_POINT('',(0.0224,-0.0285,-0.00718218971944484));
#29716=CARTESIAN_POINT('',(0.01915000000001,-0.02850000000001,-0.00718218971945484));
#29717=CARTESIAN_POINT('',(0.02715,-0.024,-0.00718218971944484));
#29718=CARTESIAN_POINT('',(0.02715000000001,-0.02400000000001,-0.00718218971945484));
#29719=CARTESIAN_POINT('',(0.01915000000001,-0.02400000000001,-0.00718218971945484));
#29720=CARTESIAN_POINT('',(0.01840000000001,-0.02285000000001,-0.00718218971945484));
#29721=CARTESIAN_POINT('',(0.02240000000001,-0.02925000000001,-0.00718218971945484));
#29722=CARTESIAN_POINT('Origin',(0.01915,-0.0285,0.00718218971944471));
#29723=CARTESIAN_POINT('',(0.02715,-0.024,0.00718218971944471));
#29724=CARTESIAN_POINT('',(0.01915000000001,-0.02400000000001,0.00718218971945471));
#29725=CARTESIAN_POINT('',(0.02715,-0.0285,0.00718218971944471));
#29726=CARTESIAN_POINT('',(0.02715000000001,-0.02850000000001,0.00718218971945471));
#29727=CARTESIAN_POINT('',(0.0224,-0.0285,0.00718218971944471));
#29728=CARTESIAN_POINT('',(0.01915000000001,-0.02850000000001,0.00718218971945471));
#29729=CARTESIAN_POINT('',(0.02240000000001,-0.02925000000001,0.00718218971945471));
#29730=CARTESIAN_POINT('',(0.01840000000001,-0.02247500000001,0.00718218971945471));
#29731=CARTESIAN_POINT('Origin',(0.0184,-0.02625,-6.57011291170234E-17));
#29732=CARTESIAN_POINT('Origin',(0.02715,-0.026625,-6.32707366852685E-17));
#29733=CARTESIAN_POINT('',(0.02715,-0.024,-0.00793218971944484));
#29734=CARTESIAN_POINT('',(0.02715000000001,-0.02400000000001,-0.00793218971945484));
#29735=CARTESIAN_POINT('',(0.02715000000001,-0.02850000000001,-0.00718218971945484));
#29736=CARTESIAN_POINT('',(0.02715,-0.024,0.00793218971944471));
#29737=CARTESIAN_POINT('',(0.02715000000001,-0.02400000000001,0.00718218971945471));
#29738=CARTESIAN_POINT('',(0.02715000000001,-0.02400000000001,0.00793218971945471));
#29739=CARTESIAN_POINT('',(0.02715000000001,-0.02925000000001,-0.00793218971945484));
#29740=CARTESIAN_POINT('Origin',(0.01915,-0.024,-0.00793218971944484));
#29741=CARTESIAN_POINT('',(0.01915000000001,-0.02400000000001,9.93506392877779E-15));
#29742=CARTESIAN_POINT('',(0.01915000000001,-0.02400000000001,-0.00793218971945484));
#29743=CARTESIAN_POINT('Origin',(0.01915,-0.024,0.00718218971944471));
#29744=CARTESIAN_POINT('',(0.01915000000001,-0.02400000000001,0.00755718971945471));
#29745=CARTESIAN_POINT('',(0.01915000000001,-0.02400000000001,0.00793218971945471));
#29746=CARTESIAN_POINT('Origin',(0.01915,-0.024,0.00793218971944471));
#29747=CARTESIAN_POINT('Origin',(0.01915,-0.02925,-0.00793218971944484));
#29748=CARTESIAN_POINT('Origin',(0.0184,-0.01645,-0.00762152954766502));
#29749=CARTESIAN_POINT('Origin',(0.01915,-0.01645,0.00793218971944471));
#29750=CARTESIAN_POINT('Origin',(0.01915,-0.0285,-0.00718218971944484));
#29751=CARTESIAN_POINT('',(0.02240000000001,-0.02850000000001,9.93612102271845E-15));
#29752=CARTESIAN_POINT('Origin',(0.0224,-0.02925,0.00718218971944471));
#34811=UNCERTAINTY_MEASURE_WITH_UNIT(LENGTH_MEASURE(1.E-5),#34877,
'DISTANCE_ACCURACY_VALUE',
'Maximum model space distance between geometric entities at asserted c
onnectivities');
#34841=UNCERTAINTY_MEASURE_WITH_UNIT(LENGTH_MEASURE(1.E-5),#34877,
'DISTANCE_ACCURACY_VALUE',
'Maximum model space distance between geometric entities at asserted c
onnectivities');
#34846=(
GEOMETRIC_REPRESENTATION_CONTEXT(3)
GLOBAL_UNCERTAINTY_ASSIGNED_CONTEXT((#34811))
GLOBAL_UNIT_ASSIGNED_CONTEXT((#34877,#34878,#34879))
REPRESENTATION_CONTEXT('','3D')
);
#34876=(
GEOMETRIC_REPRESENTATION_CONTEXT(3)
GLOBAL_UNCERTAINTY_ASSIGNED_CONTEXT((#34841))
GLOBAL_UNIT_ASSIGNED_CONTEXT((#34877,#34878,#34879))
REPRESENTATION_CONTEXT('','3D')
);
#34877=(
LENGTH_UNIT()
NAMED_UNIT(*)
SI_UNIT($,.METRE.)
);
#34878=(
NAMED_UNIT(*)
PLANE_ANGLE_UNIT()
SI_UNIT($,.RADIAN.)
);
#34879=(
NAMED_UNIT(*)
SI_UNIT($,.STERADIAN.)
SOLID_ANGLE_UNIT()
);
#34884=SHAPE_DEFINITION_REPRESENTATION(#34918,#34988);
#34918=PRODUCT_DEFINITION_SHAPE('',$,#35023);
#34988=SHAPE_REPRESENTATION('',(#20059),#34846);
#35018=PRODUCT_DEFINITION_CONTEXT('part definition',#35122,'design');
#35023=PRODUCT_DEFINITION('Motor Plastic Cover 1',
'Motor Plastic Cover 1',#35057,#35018);
#35057=PRODUCT_DEFINITION_FORMATION('',$,#35128);
#35122=APPLICATION_CONTEXT('Managed model based 3d engineering');
#35123=PRODUCT_CONTEXT('part definition',#35122,'mechanical');
#35128=PRODUCT('Motor Plastic Cover 1','Motor Plastic Cover 1',
'LEGAL AND USAGE DISCLAIMER: this Data/Model is provided \X2\201C\X0\A
S IS\X2\201D\X0\ for informational and representational only. It is a 
geometric approximation and is NOT engineered, certified, or guarantee
d for dimensional accuracy, exact tolerances, or production-level prec
ision. Vendor disclaims all implied warranties including fitness for a
 particular purpose. DO NOT USE FOR DIRECT PHYSICAL MANUFACTURING, AUT
OMATED PRODUCTION, OR SAFETY-CRITICAL SYSTEMS without independent engi
neering verification and resolution of any design discrepancies.',(#35123));
#35162=PRESENTATION_STYLE_ASSIGNMENT((#35171));
#35171=SURFACE_STYLE_USAGE(.BOTH.,#35180);
#35180=SURFACE_SIDE_STYLE('',(#35189));
#35189=SURFACE_STYLE_FILL_AREA(#35198);
#35198=FILL_AREA_STYLE('Aluminum - Anodized Glossy (Grey)',(#35207));
#35207=FILL_AREA_STYLE_COLOUR('Aluminum - Anodized Glossy (Grey)',#35216);
#35216=COLOUR_RGB('Aluminum - Anodized Glossy (Grey)',0.537254901960784,
0.537254901960784,0.537254901960784);
ENDSEC;
END-ISO-10303-21;
